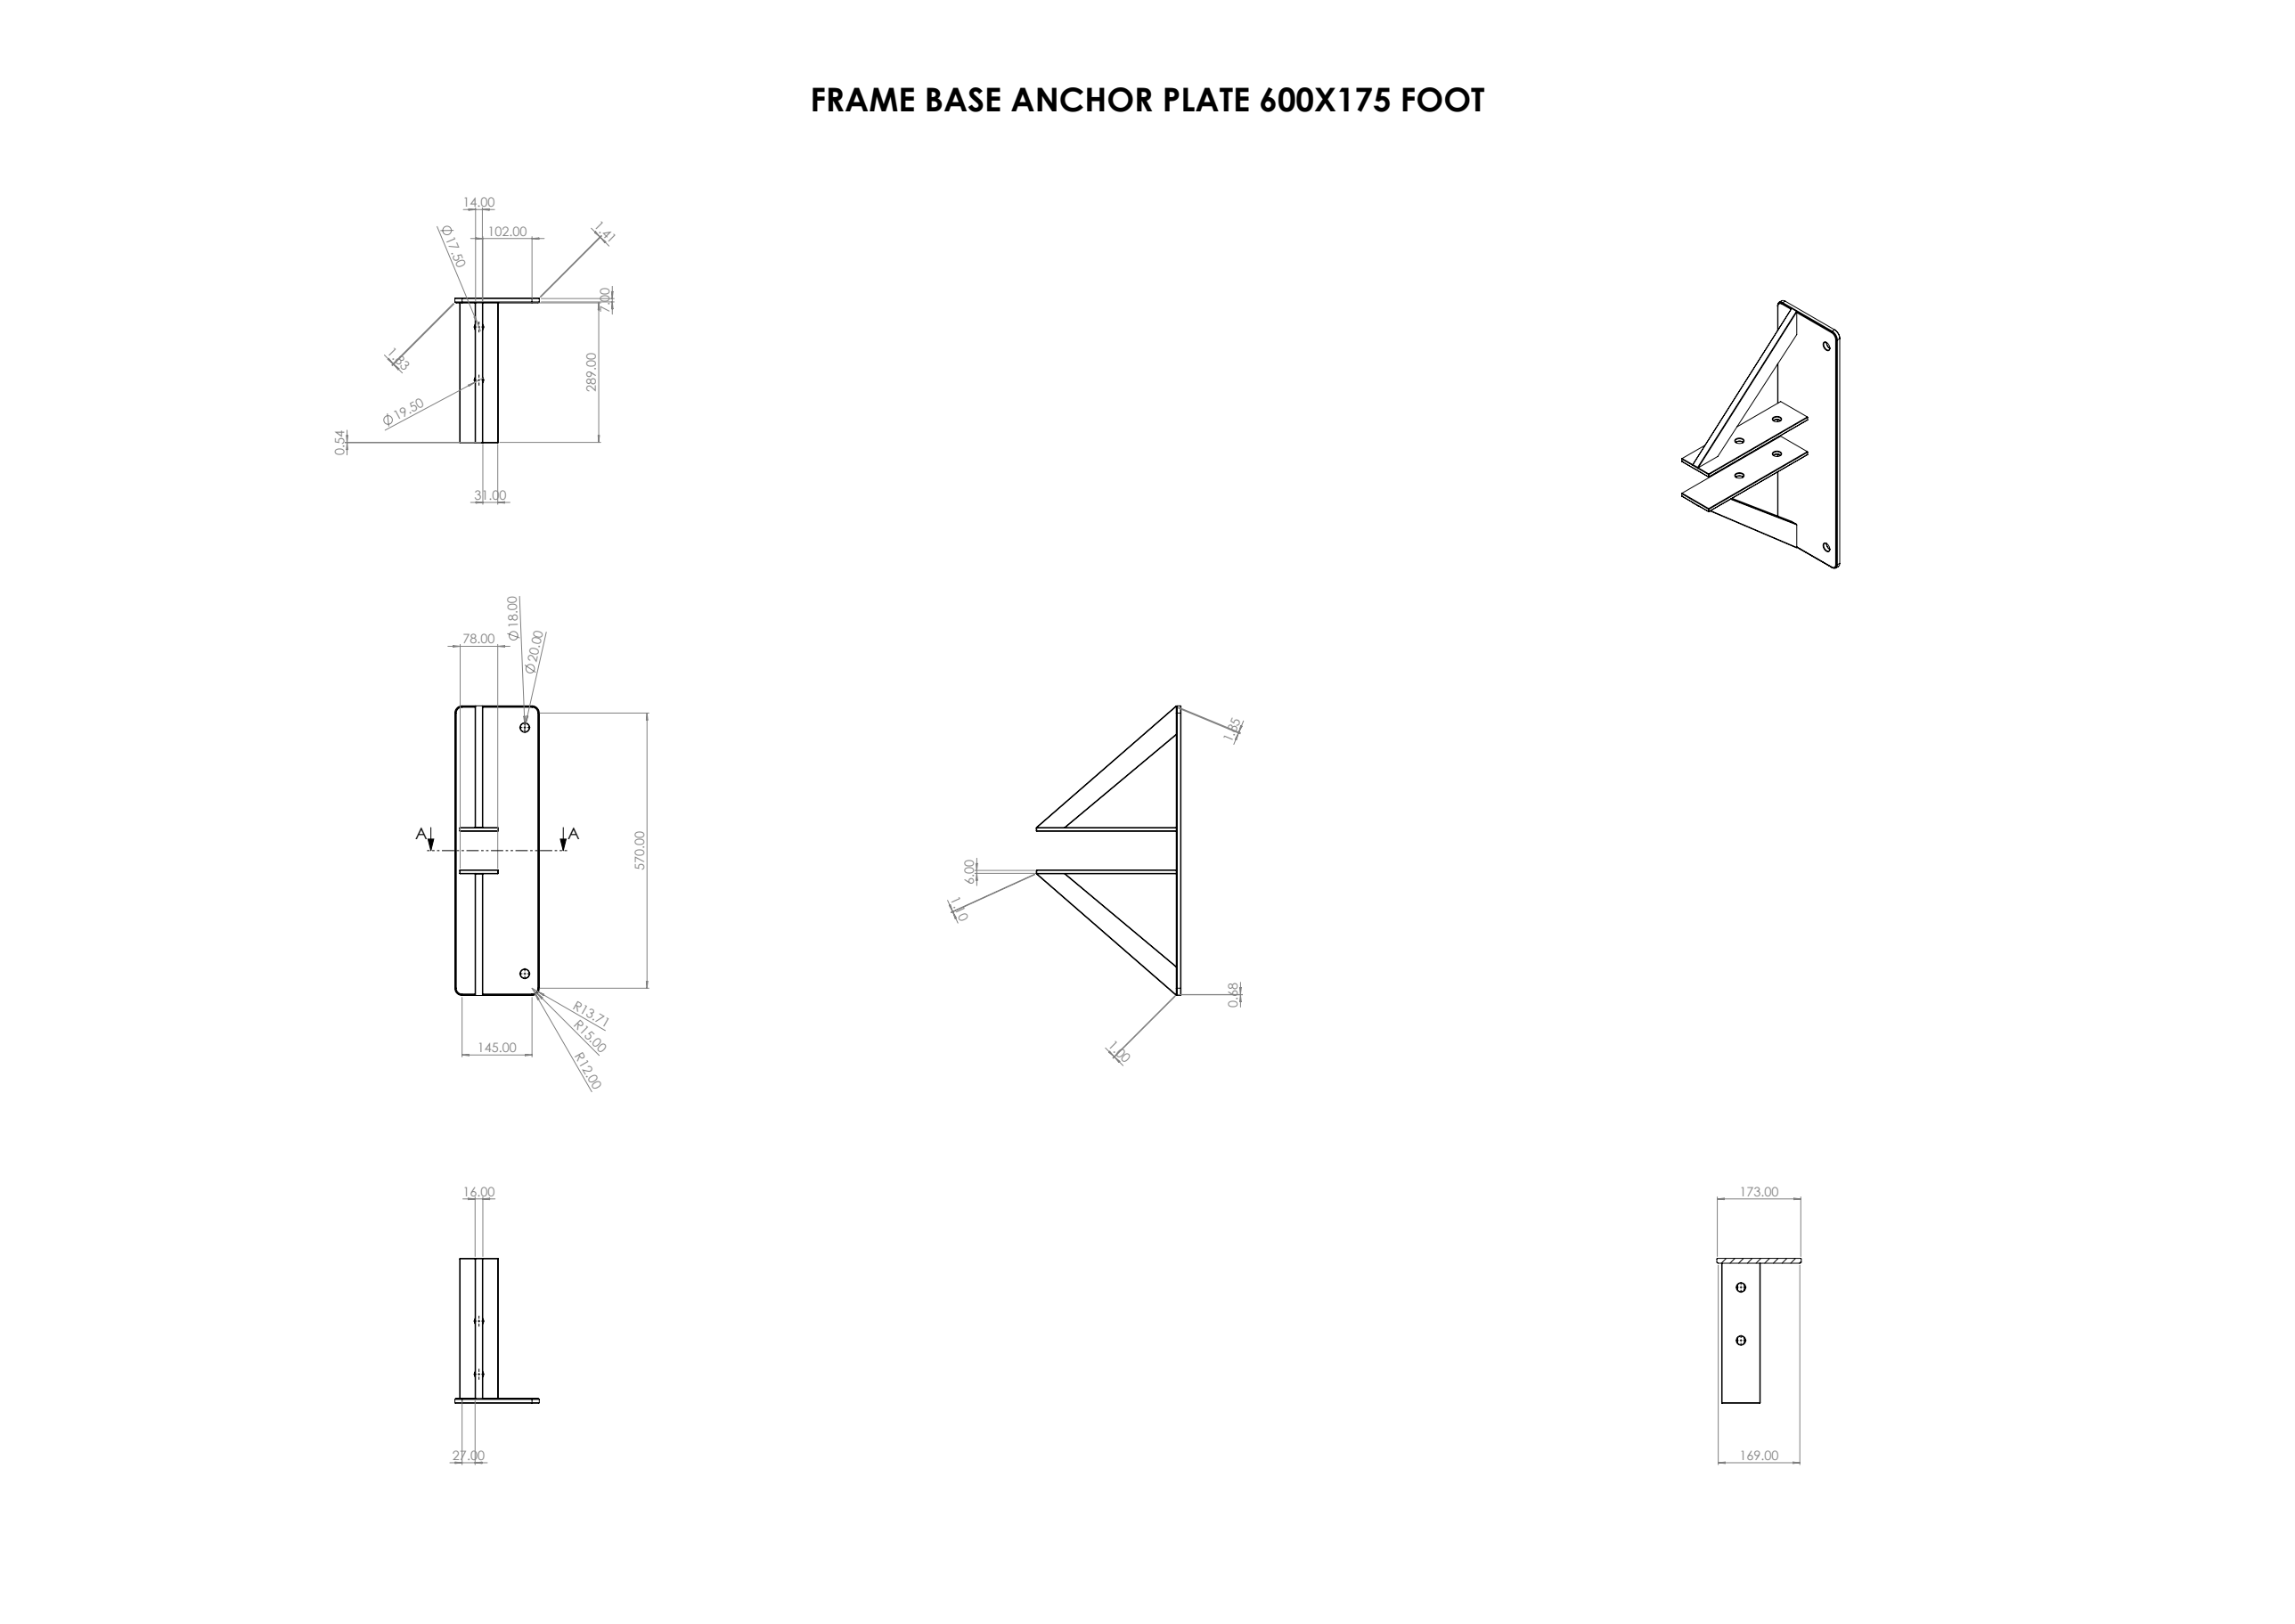
ISO-10303-21;
HEADER;
/* Generated by software containing ST-Developer
 * from STEP Tools, Inc. (www.steptools.com) 
 */

FILE_DESCRIPTION(
/* description */ (''),
/* implementation_level */ '2;1');

FILE_NAME(
/* name */ '07_Frame_Base_Anchor_Plate_600x175_Foot.step',
/* time_stamp */ '2026-10-20T10:03:03-07:00',
/* author */ (''),
/* organization */ (''),
/* preprocessor_version */ 'ST-DEVELOPER v20.2',
/* originating_system */ 'Autodesk Translation Framework v15.15.0.0',
/* authorisation */ '');

FILE_SCHEMA (('AUTOMOTIVE_DESIGN { 1 0 10303 214 3 1 1 }'));
ENDSEC;

DATA;
#10=MECHANICAL_DESIGN_GEOMETRIC_PRESENTATION_REPRESENTATION('',(#535),#71492);
#392=SHAPE_REPRESENTATION_RELATIONSHIP('SRR','None',#71613,#411);
#411=ADVANCED_BREP_SHAPE_REPRESENTATION('',(#430),#71483);
#430=MANIFOLD_SOLID_BREP('Foot',#28469);
#535=STYLED_ITEM('',(#71866),#430);
#1672=CYLINDRICAL_SURFACE('',#30065,1.5);
#1673=CYLINDRICAL_SURFACE('',#30068,1.5);
#1674=CYLINDRICAL_SURFACE('',#30093,0.875);
#1675=CYLINDRICAL_SURFACE('',#30100,0.875);
#1676=CYLINDRICAL_SURFACE('',#30108,0.875);
#1677=CYLINDRICAL_SURFACE('',#30113,0.875);
#1678=CYLINDRICAL_SURFACE('',#30118,0.899999999999999);
#1679=CYLINDRICAL_SURFACE('',#30122,0.899999999999999);
#1680=CYLINDRICAL_SURFACE('',#30161,1.5);
#1681=CYLINDRICAL_SURFACE('',#30163,1.5);
#1953=FACE_BOUND('',#5670,.T.);
#1954=FACE_BOUND('',#5671,.T.);
#1955=FACE_BOUND('',#5677,.T.);
#1956=FACE_BOUND('',#5678,.T.);
#1957=FACE_BOUND('',#5684,.T.);
#1958=FACE_BOUND('',#5685,.T.);
#1959=FACE_BOUND('',#5692,.T.);
#1960=FACE_BOUND('',#5693,.T.);
#1961=FACE_BOUND('',#5699,.T.);
#1962=FACE_BOUND('',#5700,.T.);
#1963=FACE_BOUND('',#5717,.T.);
#1964=FACE_BOUND('',#5718,.T.);
#1965=FACE_BOUND('',#5719,.T.);
#1966=FACE_BOUND('',#5720,.T.);
#2479=CIRCLE('',#30049,1.5);
#2480=CIRCLE('',#30050,1.4);
#2481=CIRCLE('',#30053,1.5);
#2482=CIRCLE('',#30054,1.4);
#2483=CIRCLE('',#30057,1.5);
#2484=CIRCLE('',#30058,1.4);
#2485=CIRCLE('',#30061,1.5);
#2486=CIRCLE('',#30062,1.4);
#2487=CIRCLE('',#30066,1.5);
#2488=CIRCLE('',#30069,1.5);
#2489=CIRCLE('',#30071,1.);
#2490=CIRCLE('',#30072,1.);
#2491=CIRCLE('',#30078,0.975000000000001);
#2492=CIRCLE('',#30079,0.975000000000001);
#2493=CIRCLE('',#30085,0.975000000000001);
#2494=CIRCLE('',#30086,0.975000000000001);
#2495=CIRCLE('',#30091,0.975000000000001);
#2496=CIRCLE('',#30092,0.875);
#2497=CIRCLE('',#30094,0.875);
#2498=CIRCLE('',#30096,0.975000000000001);
#2499=CIRCLE('',#30099,0.875);
#2500=CIRCLE('',#30101,0.875);
#2501=CIRCLE('',#30103,0.975000000000001);
#2502=CIRCLE('',#30105,0.975000000000001);
#2503=CIRCLE('',#30107,0.875);
#2504=CIRCLE('',#30109,0.875);
#2505=CIRCLE('',#30112,0.875);
#2506=CIRCLE('',#30114,0.875);
#2507=CIRCLE('',#30117,0.899999999999999);
#2508=CIRCLE('',#30119,0.899999999999999);
#2509=CIRCLE('',#30121,0.899999999999999);
#2510=CIRCLE('',#30123,0.899999999999999);
#2511=CIRCLE('',#30126,1.37071067811866);
#2512=CIRCLE('',#30127,1.2);
#2513=CIRCLE('',#30130,1.37071067811866);
#2514=CIRCLE('',#30131,1.2);
#2515=CIRCLE('',#30134,1.2);
#2516=CIRCLE('',#30135,1.2);
#2517=CIRCLE('',#30136,1.);
#2518=CIRCLE('',#30137,1.);
#2519=CIRCLE('',#30140,1.37071067811866);
#2520=CIRCLE('',#30143,1.37071067811866);
#2521=CIRCLE('',#30155,1.5);
#2522=CIRCLE('',#30158,1.5);
#2865=CONICAL_SURFACE('',#30048,1.45,0.785398163397448);
#2866=CONICAL_SURFACE('',#30052,1.45,0.78539816339746);
#2867=CONICAL_SURFACE('',#30056,1.45,0.78539816339746);
#2868=CONICAL_SURFACE('',#30060,1.45,0.785398163397448);
#2869=CONICAL_SURFACE('',#30090,0.925000000000001,0.785398163397457);
#2870=CONICAL_SURFACE('',#30097,0.925000000000001,0.785398163397457);
#2871=CONICAL_SURFACE('',#30098,0.925000000000001,0.785398163397457);
#2872=CONICAL_SURFACE('',#30102,0.925000000000001,0.785398163397457);
#2873=CONICAL_SURFACE('',#30106,0.925000000000001,0.785398163397457);
#2874=CONICAL_SURFACE('',#30110,0.925000000000001,0.785398163397457);
#2875=CONICAL_SURFACE('',#30111,0.925000000000001,0.785398163397457);
#2876=CONICAL_SURFACE('',#30115,0.925000000000001,0.785398163397457);
#2877=CONICAL_SURFACE('',#30116,0.949999999999999,0.785398163397455);
#2878=CONICAL_SURFACE('',#30120,0.949999999999999,0.785398163397455);
#2879=CONICAL_SURFACE('',#30125,1.28535533905933,1.17809724509618);
#2880=CONICAL_SURFACE('',#30129,1.28535533905933,1.17809724509618);
#2881=CONICAL_SURFACE('',#30139,1.28535533905933,1.17809724509618);
#2882=CONICAL_SURFACE('',#30142,1.28535533905933,1.17809724509618);
#2883=CONICAL_SURFACE('',#30145,0.949999999999999,0.785398163397455);
#2884=CONICAL_SURFACE('',#30146,0.949999999999999,0.785398163397455);
#2885=CONICAL_SURFACE('',#30150,1.4,0.785398163397448);
#2886=CONICAL_SURFACE('',#30152,1.4,0.785398163397448);
#2887=CONICAL_SURFACE('',#30154,1.4,0.785398163397448);
#2888=CONICAL_SURFACE('',#30157,1.4,0.785398163397448);
#3964=FACE_OUTER_BOUND('',#5623,.T.);
#3965=FACE_OUTER_BOUND('',#5624,.T.);
#3966=FACE_OUTER_BOUND('',#5625,.T.);
#3967=FACE_OUTER_BOUND('',#5626,.T.);
#3968=FACE_OUTER_BOUND('',#5627,.T.);
#3969=FACE_OUTER_BOUND('',#5628,.T.);
#3970=FACE_OUTER_BOUND('',#5629,.T.);
#3971=FACE_OUTER_BOUND('',#5630,.T.);
#3972=FACE_OUTER_BOUND('',#5631,.T.);
#3973=FACE_OUTER_BOUND('',#5632,.T.);
#3974=FACE_OUTER_BOUND('',#5633,.T.);
#3975=FACE_OUTER_BOUND('',#5634,.T.);
#3976=FACE_OUTER_BOUND('',#5635,.T.);
#3977=FACE_OUTER_BOUND('',#5636,.T.);
#3978=FACE_OUTER_BOUND('',#5637,.T.);
#3979=FACE_OUTER_BOUND('',#5638,.T.);
#3980=FACE_OUTER_BOUND('',#5639,.T.);
#3981=FACE_OUTER_BOUND('',#5640,.T.);
#3982=FACE_OUTER_BOUND('',#5641,.T.);
#3983=FACE_OUTER_BOUND('',#5642,.T.);
#3984=FACE_OUTER_BOUND('',#5643,.T.);
#3985=FACE_OUTER_BOUND('',#5644,.T.);
#3986=FACE_OUTER_BOUND('',#5645,.T.);
#3987=FACE_OUTER_BOUND('',#5646,.T.);
#3988=FACE_OUTER_BOUND('',#5647,.T.);
#3989=FACE_OUTER_BOUND('',#5648,.T.);
#3990=FACE_OUTER_BOUND('',#5649,.T.);
#3991=FACE_OUTER_BOUND('',#5650,.T.);
#3992=FACE_OUTER_BOUND('',#5651,.T.);
#3993=FACE_OUTER_BOUND('',#5652,.T.);
#3994=FACE_OUTER_BOUND('',#5653,.T.);
#3995=FACE_OUTER_BOUND('',#5654,.T.);
#3996=FACE_OUTER_BOUND('',#5655,.T.);
#3997=FACE_OUTER_BOUND('',#5656,.T.);
#3998=FACE_OUTER_BOUND('',#5657,.T.);
#3999=FACE_OUTER_BOUND('',#5658,.T.);
#4000=FACE_OUTER_BOUND('',#5659,.T.);
#4001=FACE_OUTER_BOUND('',#5660,.T.);
#4002=FACE_OUTER_BOUND('',#5661,.T.);
#4003=FACE_OUTER_BOUND('',#5662,.T.);
#4004=FACE_OUTER_BOUND('',#5663,.T.);
#4005=FACE_OUTER_BOUND('',#5664,.T.);
#4006=FACE_OUTER_BOUND('',#5665,.T.);
#4007=FACE_OUTER_BOUND('',#5666,.T.);
#4008=FACE_OUTER_BOUND('',#5667,.T.);
#4009=FACE_OUTER_BOUND('',#5668,.T.);
#4010=FACE_OUTER_BOUND('',#5669,.T.);
#4011=FACE_OUTER_BOUND('',#5672,.T.);
#4012=FACE_OUTER_BOUND('',#5673,.T.);
#4013=FACE_OUTER_BOUND('',#5674,.T.);
#4014=FACE_OUTER_BOUND('',#5675,.T.);
#4015=FACE_OUTER_BOUND('',#5676,.T.);
#4016=FACE_OUTER_BOUND('',#5679,.T.);
#4017=FACE_OUTER_BOUND('',#5680,.T.);
#4018=FACE_OUTER_BOUND('',#5681,.T.);
#4019=FACE_OUTER_BOUND('',#5682,.T.);
#4020=FACE_OUTER_BOUND('',#5683,.T.);
#4021=FACE_OUTER_BOUND('',#5686,.T.);
#4022=FACE_OUTER_BOUND('',#5687,.T.);
#4023=FACE_OUTER_BOUND('',#5688,.T.);
#4024=FACE_OUTER_BOUND('',#5689,.T.);
#4025=FACE_OUTER_BOUND('',#5690,.T.);
#4026=FACE_OUTER_BOUND('',#5691,.T.);
#4027=FACE_OUTER_BOUND('',#5694,.T.);
#4028=FACE_OUTER_BOUND('',#5695,.T.);
#4029=FACE_OUTER_BOUND('',#5696,.T.);
#4030=FACE_OUTER_BOUND('',#5697,.T.);
#4031=FACE_OUTER_BOUND('',#5698,.T.);
#4032=FACE_OUTER_BOUND('',#5701,.T.);
#4033=FACE_OUTER_BOUND('',#5702,.T.);
#4034=FACE_OUTER_BOUND('',#5703,.T.);
#4035=FACE_OUTER_BOUND('',#5704,.T.);
#4036=FACE_OUTER_BOUND('',#5705,.T.);
#4037=FACE_OUTER_BOUND('',#5706,.T.);
#4038=FACE_OUTER_BOUND('',#5707,.T.);
#4039=FACE_OUTER_BOUND('',#5708,.T.);
#4040=FACE_OUTER_BOUND('',#5709,.T.);
#4041=FACE_OUTER_BOUND('',#5710,.T.);
#4042=FACE_OUTER_BOUND('',#5711,.T.);
#4043=FACE_OUTER_BOUND('',#5712,.T.);
#4044=FACE_OUTER_BOUND('',#5713,.T.);
#4045=FACE_OUTER_BOUND('',#5714,.T.);
#4046=FACE_OUTER_BOUND('',#5715,.T.);
#4047=FACE_OUTER_BOUND('',#5716,.T.);
#4048=FACE_OUTER_BOUND('',#5721,.T.);
#4049=FACE_OUTER_BOUND('',#5722,.T.);
#4050=FACE_OUTER_BOUND('',#5723,.T.);
#4051=FACE_OUTER_BOUND('',#5724,.T.);
#4052=FACE_OUTER_BOUND('',#5725,.T.);
#4053=FACE_OUTER_BOUND('',#5726,.T.);
#4054=FACE_OUTER_BOUND('',#5727,.T.);
#4055=FACE_OUTER_BOUND('',#5728,.T.);
#4056=FACE_OUTER_BOUND('',#5729,.T.);
#4057=FACE_OUTER_BOUND('',#5730,.T.);
#4058=FACE_OUTER_BOUND('',#5731,.T.);
#4059=FACE_OUTER_BOUND('',#5732,.T.);
#4060=FACE_OUTER_BOUND('',#5733,.T.);
#4061=FACE_OUTER_BOUND('',#5734,.T.);
#4062=FACE_OUTER_BOUND('',#5735,.T.);
#4063=FACE_OUTER_BOUND('',#5736,.T.);
#4064=FACE_OUTER_BOUND('',#5737,.T.);
#4065=FACE_OUTER_BOUND('',#5738,.T.);
#4066=FACE_OUTER_BOUND('',#5739,.T.);
#4067=FACE_OUTER_BOUND('',#5740,.T.);
#4068=FACE_OUTER_BOUND('',#5741,.T.);
#4069=FACE_OUTER_BOUND('',#5742,.T.);
#5623=EDGE_LOOP('',(#23045,#23046,#23047,#23048));
#5624=EDGE_LOOP('',(#23049,#23050,#23051,#23052));
#5625=EDGE_LOOP('',(#23053,#23054,#23055,#23056));
#5626=EDGE_LOOP('',(#23057,#23058,#23059,#23060));
#5627=EDGE_LOOP('',(#23061,#23062,#23063,#23064));
#5628=EDGE_LOOP('',(#23065,#23066,#23067,#23068));
#5629=EDGE_LOOP('',(#23069,#23070,#23071,#23072,#23073));
#5630=EDGE_LOOP('',(#23074,#23075,#23076,#23077,#23078,#23079,#23080,#23081));
#5631=EDGE_LOOP('',(#23082,#23083,#23084));
#5632=EDGE_LOOP('',(#23085,#23086,#23087,#23088,#23089));
#5633=EDGE_LOOP('',(#23090,#23091,#23092));
#5634=EDGE_LOOP('',(#23093,#23094,#23095,#23096,#23097,#23098,#23099));
#5635=EDGE_LOOP('',(#23100,#23101,#23102,#23103,#23104,#23105));
#5636=EDGE_LOOP('',(#23106,#23107,#23108,#23109,#23110,#23111));
#5637=EDGE_LOOP('',(#23112,#23113,#23114,#23115,#23116,#23117));
#5638=EDGE_LOOP('',(#23118,#23119,#23120,#23121,#23122));
#5639=EDGE_LOOP('',(#23123,#23124,#23125,#23126,#23127,#23128));
#5640=EDGE_LOOP('',(#23129,#23130,#23131,#23132,#23133));
#5641=EDGE_LOOP('',(#23134,#23135,#23136,#23137,#23138));
#5642=EDGE_LOOP('',(#23139,#23140,#23141,#23142,#23143));
#5643=EDGE_LOOP('',(#23144,#23145,#23146,#23147,#23148,#23149,#23150,#23151));
#5644=EDGE_LOOP('',(#23152,#23153,#23154,#23155));
#5645=EDGE_LOOP('',(#23156,#23157,#23158,#23159,#23160,#23161,#23162));
#5646=EDGE_LOOP('',(#23163,#23164,#23165,#23166,#23167,#23168));
#5647=EDGE_LOOP('',(#23169,#23170,#23171,#23172,#23173));
#5648=EDGE_LOOP('',(#23174,#23175,#23176,#23177,#23178,#23179,#23180));
#5649=EDGE_LOOP('',(#23181,#23182,#23183));
#5650=EDGE_LOOP('',(#23184,#23185,#23186));
#5651=EDGE_LOOP('',(#23187,#23188,#23189,#23190,#23191,#23192));
#5652=EDGE_LOOP('',(#23193,#23194,#23195,#23196,#23197,#23198));
#5653=EDGE_LOOP('',(#23199,#23200,#23201,#23202,#23203));
#5654=EDGE_LOOP('',(#23204,#23205,#23206,#23207,#23208,#23209));
#5655=EDGE_LOOP('',(#23210,#23211,#23212,#23213,#23214,#23215));
#5656=EDGE_LOOP('',(#23216,#23217,#23218,#23219,#23220));
#5657=EDGE_LOOP('',(#23221,#23222,#23223,#23224));
#5658=EDGE_LOOP('',(#23225,#23226,#23227,#23228));
#5659=EDGE_LOOP('',(#23229,#23230,#23231,#23232));
#5660=EDGE_LOOP('',(#23233,#23234,#23235,#23236));
#5661=EDGE_LOOP('',(#23237,#23238,#23239,#23240));
#5662=EDGE_LOOP('',(#23241,#23242,#23243,#23244));
#5663=EDGE_LOOP('',(#23245,#23246,#23247,#23248));
#5664=EDGE_LOOP('',(#23249,#23250,#23251,#23252));
#5665=EDGE_LOOP('',(#23253,#23254,#23255,#23256));
#5666=EDGE_LOOP('',(#23257,#23258,#23259,#23260));
#5667=EDGE_LOOP('',(#23261,#23262,#23263,#23264));
#5668=EDGE_LOOP('',(#23265,#23266,#23267,#23268));
#5669=EDGE_LOOP('',(#23269,#23270,#23271,#23272,#23273,#23274,#23275,#23276));
#5670=EDGE_LOOP('',(#23277));
#5671=EDGE_LOOP('',(#23278));
#5672=EDGE_LOOP('',(#23279,#23280,#23281,#23282));
#5673=EDGE_LOOP('',(#23283,#23284,#23285,#23286));
#5674=EDGE_LOOP('',(#23287,#23288,#23289,#23290,#23291));
#5675=EDGE_LOOP('',(#23292,#23293,#23294,#23295,#23296));
#5676=EDGE_LOOP('',(#23297,#23298,#23299,#23300,#23301,#23302,#23303,#23304,
#23305,#23306,#23307,#23308,#23309,#23310,#23311,#23312));
#5677=EDGE_LOOP('',(#23313));
#5678=EDGE_LOOP('',(#23314));
#5679=EDGE_LOOP('',(#23315,#23316,#23317,#23318,#23319));
#5680=EDGE_LOOP('',(#23320,#23321,#23322,#23323,#23324));
#5681=EDGE_LOOP('',(#23325,#23326,#23327,#23328,#23329));
#5682=EDGE_LOOP('',(#23330,#23331,#23332,#23333,#23334));
#5683=EDGE_LOOP('',(#23335,#23336,#23337,#23338,#23339,#23340,#23341,#23342,
#23343,#23344,#23345,#23346,#23347,#23348,#23349,#23350));
#5684=EDGE_LOOP('',(#23351));
#5685=EDGE_LOOP('',(#23352));
#5686=EDGE_LOOP('',(#23353,#23354,#23355,#23356));
#5687=EDGE_LOOP('',(#23357,#23358,#23359,#23360,#23361));
#5688=EDGE_LOOP('',(#23362,#23363,#23364,#23365));
#5689=EDGE_LOOP('',(#23366,#23367,#23368,#23369));
#5690=EDGE_LOOP('',(#23370,#23371,#23372,#23373));
#5691=EDGE_LOOP('',(#23374,#23375,#23376,#23377));
#5692=EDGE_LOOP('',(#23378));
#5693=EDGE_LOOP('',(#23379));
#5694=EDGE_LOOP('',(#23380,#23381,#23382,#23383));
#5695=EDGE_LOOP('',(#23384,#23385,#23386,#23387));
#5696=EDGE_LOOP('',(#23388,#23389,#23390,#23391));
#5697=EDGE_LOOP('',(#23392,#23393,#23394,#23395));
#5698=EDGE_LOOP('',(#23396,#23397,#23398,#23399));
#5699=EDGE_LOOP('',(#23400));
#5700=EDGE_LOOP('',(#23401));
#5701=EDGE_LOOP('',(#23402,#23403,#23404,#23405));
#5702=EDGE_LOOP('',(#23406,#23407,#23408,#23409));
#5703=EDGE_LOOP('',(#23410,#23411,#23412,#23413));
#5704=EDGE_LOOP('',(#23414,#23415,#23416,#23417));
#5705=EDGE_LOOP('',(#23418,#23419,#23420,#23421));
#5706=EDGE_LOOP('',(#23422,#23423,#23424,#23425));
#5707=EDGE_LOOP('',(#23426,#23427,#23428,#23429));
#5708=EDGE_LOOP('',(#23430,#23431,#23432,#23433));
#5709=EDGE_LOOP('',(#23434,#23435,#23436,#23437));
#5710=EDGE_LOOP('',(#23438,#23439,#23440,#23441));
#5711=EDGE_LOOP('',(#23442,#23443,#23444,#23445));
#5712=EDGE_LOOP('',(#23446,#23447,#23448,#23449));
#5713=EDGE_LOOP('',(#23450,#23451,#23452,#23453));
#5714=EDGE_LOOP('',(#23454,#23455,#23456,#23457));
#5715=EDGE_LOOP('',(#23458,#23459,#23460,#23461));
#5716=EDGE_LOOP('',(#23462,#23463,#23464,#23465,#23466,#23467,#23468,#23469,
#23470,#23471,#23472,#23473,#23474,#23475,#23476,#23477,#23478,#23479,#23480,
#23481));
#5717=EDGE_LOOP('',(#23482));
#5718=EDGE_LOOP('',(#23483,#23484,#23485,#23486,#23487,#23488,#23489,#23490));
#5719=EDGE_LOOP('',(#23491,#23492,#23493,#23494,#23495,#23496,#23497,#23498));
#5720=EDGE_LOOP('',(#23499));
#5721=EDGE_LOOP('',(#23500,#23501,#23502,#23503));
#5722=EDGE_LOOP('',(#23504,#23505,#23506,#23507));
#5723=EDGE_LOOP('',(#23508,#23509,#23510,#23511));
#5724=EDGE_LOOP('',(#23512,#23513,#23514,#23515));
#5725=EDGE_LOOP('',(#23516,#23517,#23518,#23519));
#5726=EDGE_LOOP('',(#23520,#23521,#23522,#23523));
#5727=EDGE_LOOP('',(#23524,#23525,#23526,#23527));
#5728=EDGE_LOOP('',(#23528,#23529,#23530,#23531));
#5729=EDGE_LOOP('',(#23532,#23533,#23534,#23535,#23536,#23537));
#5730=EDGE_LOOP('',(#23538,#23539,#23540,#23541,#23542,#23543,#23544));
#5731=EDGE_LOOP('',(#23545,#23546,#23547,#23548));
#5732=EDGE_LOOP('',(#23549,#23550,#23551,#23552));
#5733=EDGE_LOOP('',(#23553,#23554,#23555,#23556));
#5734=EDGE_LOOP('',(#23557,#23558,#23559,#23560,#23561,#23562,#23563,#23564));
#5735=EDGE_LOOP('',(#23565,#23566,#23567,#23568));
#5736=EDGE_LOOP('',(#23569,#23570,#23571,#23572));
#5737=EDGE_LOOP('',(#23573,#23574,#23575,#23576));
#5738=EDGE_LOOP('',(#23577,#23578,#23579,#23580,#23581,#23582,#23583,#23584));
#5739=EDGE_LOOP('',(#23585,#23586,#23587,#23588));
#5740=EDGE_LOOP('',(#23589,#23590,#23591,#23592));
#5741=EDGE_LOOP('',(#23593,#23594,#23595,#23596));
#5742=EDGE_LOOP('',(#23597,#23598,#23599,#23600));
#8008=LINE('',#50006,#10496);
#8009=LINE('',#50008,#10497);
#8010=LINE('',#50010,#10498);
#8011=LINE('',#50011,#10499);
#8012=LINE('',#50014,#10500);
#8013=LINE('',#50016,#10501);
#8014=LINE('',#50017,#10502);
#8015=LINE('',#50020,#10503);
#8016=LINE('',#50022,#10504);
#8017=LINE('',#50023,#10505);
#8018=LINE('',#50027,#10506);
#8019=LINE('',#50029,#10507);
#8020=LINE('',#50031,#10508);
#8021=LINE('',#50032,#10509);
#8022=LINE('',#50035,#10510);
#8023=LINE('',#50037,#10511);
#8024=LINE('',#50038,#10512);
#8025=LINE('',#50041,#10513);
#8026=LINE('',#50043,#10514);
#8027=LINE('',#50044,#10515);
#8028=LINE('',#50048,#10516);
#8029=LINE('',#50050,#10517);
#8030=LINE('',#50052,#10518);
#8031=LINE('',#50054,#10519);
#8032=LINE('',#50055,#10520);
#8033=LINE('',#50058,#10521);
#8034=LINE('',#50060,#10522);
#8035=LINE('',#50062,#10523);
#8036=LINE('',#50064,#10524);
#8037=LINE('',#50066,#10525);
#8038=LINE('',#50068,#10526);
#8039=LINE('',#50069,#10527);
#8040=LINE('',#50072,#10528);
#8041=LINE('',#50073,#10529);
#8042=LINE('',#50076,#10530);
#8043=LINE('',#50078,#10531);
#8044=LINE('',#50080,#10532);
#8045=LINE('',#50081,#10533);
#8046=LINE('',#50084,#10534);
#8047=LINE('',#50085,#10535);
#8048=LINE('',#50088,#10536);
#8049=LINE('',#50090,#10537);
#8050=LINE('',#50092,#10538);
#8051=LINE('',#50093,#10539);
#8052=LINE('',#50094,#10540);
#8053=LINE('',#50097,#10541);
#8054=LINE('',#50099,#10542);
#8055=LINE('',#50101,#10543);
#8056=LINE('',#50103,#10544);
#8057=LINE('',#50104,#10545);
#8058=LINE('',#50107,#10546);
#8059=LINE('',#50109,#10547);
#8060=LINE('',#50111,#10548);
#8061=LINE('',#50113,#10549);
#8062=LINE('',#50114,#10550);
#8063=LINE('',#50117,#10551);
#8064=LINE('',#50119,#10552);
#8065=LINE('',#50121,#10553);
#8066=LINE('',#50122,#10554);
#8067=LINE('',#50125,#10555);
#8068=LINE('',#50127,#10556);
#8069=LINE('',#50128,#10557);
#8070=LINE('',#50131,#10558);
#8071=LINE('',#50133,#10559);
#8072=LINE('',#50135,#10560);
#8073=LINE('',#50136,#10561);
#8074=LINE('',#50139,#10562);
#8075=LINE('',#50140,#10563);
#8076=LINE('',#50143,#10564);
#8077=LINE('',#50145,#10565);
#8078=LINE('',#50146,#10566);
#8079=LINE('',#50150,#10567);
#8080=LINE('',#50152,#10568);
#8081=LINE('',#50154,#10569);
#8082=LINE('',#50156,#10570);
#8083=LINE('',#50157,#10571);
#8084=LINE('',#50160,#10572);
#8085=LINE('',#50162,#10573);
#8086=LINE('',#50164,#10574);
#8087=LINE('',#50166,#10575);
#8088=LINE('',#50168,#10576);
#8089=LINE('',#50170,#10577);
#8090=LINE('',#50171,#10578);
#8091=LINE('',#50174,#10579);
#8092=LINE('',#50175,#10580);
#8093=LINE('',#50178,#10581);
#8094=LINE('',#50180,#10582);
#8095=LINE('',#50182,#10583);
#8096=LINE('',#50183,#10584);
#8097=LINE('',#50184,#10585);
#8098=LINE('',#50187,#10586);
#8099=LINE('',#50189,#10587);
#8100=LINE('',#50190,#10588);
#8101=LINE('',#50193,#10589);
#8102=LINE('',#50194,#10590);
#8103=LINE('',#50196,#10591);
#8104=LINE('',#50198,#10592);
#8105=LINE('',#50200,#10593);
#8106=LINE('',#50201,#10594);
#8107=LINE('',#50204,#10595);
#8108=LINE('',#50205,#10596);
#8109=LINE('',#50208,#10597);
#8110=LINE('',#50209,#10598);
#8111=LINE('',#50212,#10599);
#8112=LINE('',#50214,#10600);
#8113=LINE('',#50216,#10601);
#8114=LINE('',#50218,#10602);
#8115=LINE('',#50219,#10603);
#8116=LINE('',#50222,#10604);
#8117=LINE('',#50224,#10605);
#8118=LINE('',#50226,#10606);
#8119=LINE('',#50228,#10607);
#8120=LINE('',#50229,#10608);
#8121=LINE('',#50232,#10609);
#8122=LINE('',#50234,#10610);
#8123=LINE('',#50236,#10611);
#8124=LINE('',#50237,#10612);
#8125=LINE('',#50240,#10613);
#8126=LINE('',#50242,#10614);
#8127=LINE('',#50243,#10615);
#8128=LINE('',#50246,#10616);
#8129=LINE('',#50248,#10617);
#8130=LINE('',#50250,#10618);
#8131=LINE('',#50251,#10619);
#8132=LINE('',#50254,#10620);
#8133=LINE('',#50256,#10621);
#8134=LINE('',#50257,#10622);
#8135=LINE('',#50261,#10623);
#8136=LINE('',#50265,#10624);
#8137=LINE('',#50270,#10625);
#8138=LINE('',#50271,#10626);
#8139=LINE('',#50272,#10627);
#8140=LINE('',#50276,#10628);
#8141=LINE('',#50282,#10629);
#8142=LINE('',#50283,#10630);
#8143=LINE('',#50284,#10631);
#8144=LINE('',#50288,#10632);
#8145=LINE('',#50294,#10633);
#8146=LINE('',#50295,#10634);
#8147=LINE('',#50296,#10635);
#8148=LINE('',#50300,#10636);
#8149=LINE('',#50304,#10637);
#8150=LINE('',#50305,#10638);
#8151=LINE('',#50308,#10639);
#8152=LINE('',#50310,#10640);
#8153=LINE('',#50311,#10641);
#8154=LINE('',#50314,#10642);
#8155=LINE('',#50318,#10643);
#8156=LINE('',#50319,#10644);
#8157=LINE('',#50322,#10645);
#8158=LINE('',#50331,#10646);
#8159=LINE('',#50332,#10647);
#8160=LINE('',#50335,#10648);
#8161=LINE('',#50336,#10649);
#8162=LINE('',#50339,#10650);
#8163=LINE('',#50341,#10651);
#8164=LINE('',#50342,#10652);
#8165=LINE('',#50344,#10653);
#8166=LINE('',#50347,#10654);
#8167=LINE('',#50349,#10655);
#8168=LINE('',#50350,#10656);
#8169=LINE('',#50356,#10657);
#8170=LINE('',#50357,#10658);
#8171=LINE('',#50361,#10659);
#8172=LINE('',#50363,#10660);
#8173=LINE('',#50365,#10661);
#8174=LINE('',#50366,#10662);
#8175=LINE('',#50368,#10663);
#8176=LINE('',#50370,#10664);
#8177=LINE('',#50371,#10665);
#8178=LINE('',#50378,#10666);
#8179=LINE('',#50379,#10667);
#8180=LINE('',#50382,#10668);
#8181=LINE('',#50383,#10669);
#8182=LINE('',#50385,#10670);
#8183=LINE('',#50390,#10671);
#8184=LINE('',#50395,#10672);
#8185=LINE('',#50397,#10673);
#8186=LINE('',#50401,#10674);
#8187=LINE('',#50404,#10675);
#8188=LINE('',#50409,#10676);
#8189=LINE('',#50413,#10677);
#8190=LINE('',#50415,#10678);
#8191=LINE('',#50420,#10679);
#8192=LINE('',#50425,#10680);
#8193=LINE('',#50427,#10681);
#8194=LINE('',#50430,#10682);
#8195=LINE('',#50435,#10683);
#8196=LINE('',#50437,#10684);
#8197=LINE('',#50440,#10685);
#8198=LINE('',#50444,#10686);
#8199=LINE('',#50448,#10687);
#8200=LINE('',#50452,#10688);
#8201=LINE('',#50456,#10689);
#8202=LINE('',#50458,#10690);
#8203=LINE('',#50459,#10691);
#8204=LINE('',#50463,#10692);
#8205=LINE('',#50469,#10693);
#8206=LINE('',#50470,#10694);
#8207=LINE('',#50471,#10695);
#8208=LINE('',#50475,#10696);
#8209=LINE('',#50479,#10697);
#8210=LINE('',#50480,#10698);
#8211=LINE('',#50483,#10699);
#8212=LINE('',#50485,#10700);
#8213=LINE('',#50489,#10701);
#8214=LINE('',#50492,#10702);
#8215=LINE('',#50499,#10703);
#8216=LINE('',#50500,#10704);
#8217=LINE('',#50503,#10705);
#8218=LINE('',#50507,#10706);
#8219=LINE('',#50508,#10707);
#8220=LINE('',#50511,#10708);
#8221=LINE('',#50515,#10709);
#8222=LINE('',#50516,#10710);
#8223=LINE('',#50518,#10711);
#8224=LINE('',#50520,#10712);
#8225=LINE('',#50522,#10713);
#8226=LINE('',#50525,#10714);
#8227=LINE('',#50526,#10715);
#8228=LINE('',#50528,#10716);
#8229=LINE('',#50530,#10717);
#8230=LINE('',#50531,#10718);
#8231=LINE('',#50533,#10719);
#8232=LINE('',#50535,#10720);
#8233=LINE('',#50537,#10721);
#8234=LINE('',#50540,#10722);
#8235=LINE('',#50544,#10723);
#8236=LINE('',#50545,#10724);
#8237=LINE('',#50548,#10725);
#8238=LINE('',#50551,#10726);
#8239=LINE('',#50553,#10727);
#8240=LINE('',#50554,#10728);
#8241=LINE('',#50556,#10729);
#10496=VECTOR('',#35215,1.);
#10497=VECTOR('',#35216,1.);
#10498=VECTOR('',#35217,1.);
#10499=VECTOR('',#35218,1.);
#10500=VECTOR('',#35221,1.);
#10501=VECTOR('',#35222,1.);
#10502=VECTOR('',#35223,1.);
#10503=VECTOR('',#35226,1.);
#10504=VECTOR('',#35227,1.);
#10505=VECTOR('',#35228,1.);
#10506=VECTOR('',#35231,1.);
#10507=VECTOR('',#35232,1.);
#10508=VECTOR('',#35233,1.);
#10509=VECTOR('',#35234,1.);
#10510=VECTOR('',#35237,1.);
#10511=VECTOR('',#35238,1.);
#10512=VECTOR('',#35239,1.);
#10513=VECTOR('',#35242,1.);
#10514=VECTOR('',#35243,1.);
#10515=VECTOR('',#35244,1.);
#10516=VECTOR('',#35247,1.);
#10517=VECTOR('',#35248,1.);
#10518=VECTOR('',#35249,1.);
#10519=VECTOR('',#35250,1.);
#10520=VECTOR('',#35251,1.);
#10521=VECTOR('',#35254,1.);
#10522=VECTOR('',#35255,1.);
#10523=VECTOR('',#35256,1.);
#10524=VECTOR('',#35257,1.);
#10525=VECTOR('',#35258,1.);
#10526=VECTOR('',#35259,1.);
#10527=VECTOR('',#35260,1.);
#10528=VECTOR('',#35263,1.);
#10529=VECTOR('',#35264,1.);
#10530=VECTOR('',#35267,1.);
#10531=VECTOR('',#35268,1.);
#10532=VECTOR('',#35269,1.);
#10533=VECTOR('',#35270,1.);
#10534=VECTOR('',#35273,1.);
#10535=VECTOR('',#35274,1.);
#10536=VECTOR('',#35277,1.);
#10537=VECTOR('',#35278,1.);
#10538=VECTOR('',#35279,1.);
#10539=VECTOR('',#35280,1.);
#10540=VECTOR('',#35281,1.);
#10541=VECTOR('',#35284,1.);
#10542=VECTOR('',#35285,1.);
#10543=VECTOR('',#35286,1.);
#10544=VECTOR('',#35287,1.);
#10545=VECTOR('',#35288,1.);
#10546=VECTOR('',#35291,1.);
#10547=VECTOR('',#35292,1.);
#10548=VECTOR('',#35293,1.);
#10549=VECTOR('',#35294,1.);
#10550=VECTOR('',#35295,1.);
#10551=VECTOR('',#35298,1.);
#10552=VECTOR('',#35299,1.);
#10553=VECTOR('',#35300,1.);
#10554=VECTOR('',#35301,1.);
#10555=VECTOR('',#35304,1.);
#10556=VECTOR('',#35305,1.);
#10557=VECTOR('',#35306,1.);
#10558=VECTOR('',#35309,1.);
#10559=VECTOR('',#35310,1.);
#10560=VECTOR('',#35311,1.);
#10561=VECTOR('',#35312,1.);
#10562=VECTOR('',#35315,1.);
#10563=VECTOR('',#35316,1.);
#10564=VECTOR('',#35319,1.);
#10565=VECTOR('',#35320,1.);
#10566=VECTOR('',#35321,1.);
#10567=VECTOR('',#35324,1.);
#10568=VECTOR('',#35325,1.);
#10569=VECTOR('',#35326,1.);
#10570=VECTOR('',#35327,1.);
#10571=VECTOR('',#35328,1.);
#10572=VECTOR('',#35331,1.);
#10573=VECTOR('',#35332,1.);
#10574=VECTOR('',#35333,1.);
#10575=VECTOR('',#35334,1.);
#10576=VECTOR('',#35335,1.);
#10577=VECTOR('',#35336,1.);
#10578=VECTOR('',#35337,1.);
#10579=VECTOR('',#35340,1.);
#10580=VECTOR('',#35341,1.);
#10581=VECTOR('',#35344,1.);
#10582=VECTOR('',#35345,1.);
#10583=VECTOR('',#35346,1.);
#10584=VECTOR('',#35347,1.);
#10585=VECTOR('',#35348,1.);
#10586=VECTOR('',#35351,1.);
#10587=VECTOR('',#35352,1.);
#10588=VECTOR('',#35353,1.);
#10589=VECTOR('',#35356,1.);
#10590=VECTOR('',#35357,1.);
#10591=VECTOR('',#35360,1.);
#10592=VECTOR('',#35361,1.);
#10593=VECTOR('',#35362,1.);
#10594=VECTOR('',#35363,1.);
#10595=VECTOR('',#35366,1.);
#10596=VECTOR('',#35367,1.);
#10597=VECTOR('',#35370,1.);
#10598=VECTOR('',#35371,1.);
#10599=VECTOR('',#35374,1.);
#10600=VECTOR('',#35375,1.);
#10601=VECTOR('',#35376,1.);
#10602=VECTOR('',#35377,1.);
#10603=VECTOR('',#35378,1.);
#10604=VECTOR('',#35381,1.);
#10605=VECTOR('',#35382,1.);
#10606=VECTOR('',#35383,1.);
#10607=VECTOR('',#35384,1.);
#10608=VECTOR('',#35385,1.);
#10609=VECTOR('',#35388,1.);
#10610=VECTOR('',#35389,1.);
#10611=VECTOR('',#35390,1.);
#10612=VECTOR('',#35391,1.);
#10613=VECTOR('',#35394,1.);
#10614=VECTOR('',#35395,1.);
#10615=VECTOR('',#35396,1.);
#10616=VECTOR('',#35399,1.);
#10617=VECTOR('',#35400,1.);
#10618=VECTOR('',#35401,1.);
#10619=VECTOR('',#35402,1.);
#10620=VECTOR('',#35405,1.);
#10621=VECTOR('',#35406,1.);
#10622=VECTOR('',#35407,1.);
#10623=VECTOR('',#35410,1.);
#10624=VECTOR('',#35413,1.);
#10625=VECTOR('',#35418,1.);
#10626=VECTOR('',#35419,1.);
#10627=VECTOR('',#35420,1.);
#10628=VECTOR('',#35423,1.);
#10629=VECTOR('',#35430,1.);
#10630=VECTOR('',#35431,1.);
#10631=VECTOR('',#35432,1.);
#10632=VECTOR('',#35435,1.);
#10633=VECTOR('',#35442,1.);
#10634=VECTOR('',#35443,1.);
#10635=VECTOR('',#35444,1.);
#10636=VECTOR('',#35447,1.);
#10637=VECTOR('',#35454,1.);
#10638=VECTOR('',#35455,1.);
#10639=VECTOR('',#35458,1.);
#10640=VECTOR('',#35459,1.);
#10641=VECTOR('',#35460,1.);
#10642=VECTOR('',#35463,1.);
#10643=VECTOR('',#35468,1.);
#10644=VECTOR('',#35469,1.);
#10645=VECTOR('',#35472,1.);
#10646=VECTOR('',#35483,1.);
#10647=VECTOR('',#35484,1.);
#10648=VECTOR('',#35487,1.);
#10649=VECTOR('',#35488,1.);
#10650=VECTOR('',#35491,1.);
#10651=VECTOR('',#35492,1.);
#10652=VECTOR('',#35493,1.);
#10653=VECTOR('',#35496,1.);
#10654=VECTOR('',#35499,1.);
#10655=VECTOR('',#35500,1.);
#10656=VECTOR('',#35501,1.);
#10657=VECTOR('',#35508,1.);
#10658=VECTOR('',#35509,1.);
#10659=VECTOR('',#35514,1.);
#10660=VECTOR('',#35515,1.);
#10661=VECTOR('',#35516,1.);
#10662=VECTOR('',#35517,1.);
#10663=VECTOR('',#35520,1.);
#10664=VECTOR('',#35523,1.);
#10665=VECTOR('',#35524,1.);
#10666=VECTOR('',#35531,1.);
#10667=VECTOR('',#35532,1.);
#10668=VECTOR('',#35535,1.);
#10669=VECTOR('',#35536,1.);
#10670=VECTOR('',#35539,1.);
#10671=VECTOR('',#35544,0.925000000000001);
#10672=VECTOR('',#35551,0.875);
#10673=VECTOR('',#35554,1.);
#10674=VECTOR('',#35559,0.925000000000001);
#10675=VECTOR('',#35562,0.925000000000001);
#10676=VECTOR('',#35569,0.875);
#10677=VECTOR('',#35574,0.925000000000001);
#10678=VECTOR('',#35577,1.);
#10679=VECTOR('',#35582,0.925000000000001);
#10680=VECTOR('',#35589,0.875);
#10681=VECTOR('',#35592,0.925000000000001);
#10682=VECTOR('',#35595,0.925000000000001);
#10683=VECTOR('',#35602,0.875);
#10684=VECTOR('',#35605,0.925000000000001);
#10685=VECTOR('',#35608,0.949999999999999);
#10686=VECTOR('',#35613,0.899999999999999);
#10687=VECTOR('',#35618,0.949999999999999);
#10688=VECTOR('',#35623,0.899999999999999);
#10689=VECTOR('',#35628,1.);
#10690=VECTOR('',#35629,1.);
#10691=VECTOR('',#35630,1.);
#10692=VECTOR('',#35633,1.);
#10693=VECTOR('',#35640,1.);
#10694=VECTOR('',#35641,1.);
#10695=VECTOR('',#35642,1.);
#10696=VECTOR('',#35645,1.);
#10697=VECTOR('',#35652,1.);
#10698=VECTOR('',#35653,1.);
#10699=VECTOR('',#35656,1.);
#10700=VECTOR('',#35657,1.);
#10701=VECTOR('',#35660,1.);
#10702=VECTOR('',#35663,1.);
#10703=VECTOR('',#35670,1.);
#10704=VECTOR('',#35671,1.);
#10705=VECTOR('',#35674,1.);
#10706=VECTOR('',#35679,1.);
#10707=VECTOR('',#35680,1.);
#10708=VECTOR('',#35683,1.);
#10709=VECTOR('',#35688,1.);
#10710=VECTOR('',#35689,1.);
#10711=VECTOR('',#35692,0.949999999999999);
#10712=VECTOR('',#35695,0.949999999999999);
#10713=VECTOR('',#35698,1.);
#10714=VECTOR('',#35701,1.);
#10715=VECTOR('',#35702,1.);
#10716=VECTOR('',#35705,1.);
#10717=VECTOR('',#35708,1.);
#10718=VECTOR('',#35709,1.);
#10719=VECTOR('',#35712,1.);
#10720=VECTOR('',#35715,1.);
#10721=VECTOR('',#35718,1.);
#10722=VECTOR('',#35721,1.);
#10723=VECTOR('',#35726,1.);
#10724=VECTOR('',#35727,1.);
#10725=VECTOR('',#35730,1.);
#10726=VECTOR('',#35735,1.);
#10727=VECTOR('',#35738,1.);
#10728=VECTOR('',#35739,1.);
#10729=VECTOR('',#35742,1.);
#12885=VERTEX_POINT('',#50004);
#12886=VERTEX_POINT('',#50005);
#12887=VERTEX_POINT('',#50007);
#12888=VERTEX_POINT('',#50009);
#12889=VERTEX_POINT('',#50013);
#12890=VERTEX_POINT('',#50015);
#12891=VERTEX_POINT('',#50019);
#12892=VERTEX_POINT('',#50021);
#12893=VERTEX_POINT('',#50025);
#12894=VERTEX_POINT('',#50026);
#12895=VERTEX_POINT('',#50028);
#12896=VERTEX_POINT('',#50030);
#12897=VERTEX_POINT('',#50034);
#12898=VERTEX_POINT('',#50036);
#12899=VERTEX_POINT('',#50040);
#12900=VERTEX_POINT('',#50042);
#12901=VERTEX_POINT('',#50046);
#12902=VERTEX_POINT('',#50047);
#12903=VERTEX_POINT('',#50049);
#12904=VERTEX_POINT('',#50051);
#12905=VERTEX_POINT('',#50053);
#12906=VERTEX_POINT('',#50057);
#12907=VERTEX_POINT('',#50059);
#12908=VERTEX_POINT('',#50061);
#12909=VERTEX_POINT('',#50063);
#12910=VERTEX_POINT('',#50065);
#12911=VERTEX_POINT('',#50067);
#12912=VERTEX_POINT('',#50071);
#12913=VERTEX_POINT('',#50075);
#12914=VERTEX_POINT('',#50077);
#12915=VERTEX_POINT('',#50079);
#12916=VERTEX_POINT('',#50083);
#12917=VERTEX_POINT('',#50087);
#12918=VERTEX_POINT('',#50089);
#12919=VERTEX_POINT('',#50091);
#12920=VERTEX_POINT('',#50096);
#12921=VERTEX_POINT('',#50098);
#12922=VERTEX_POINT('',#50100);
#12923=VERTEX_POINT('',#50102);
#12924=VERTEX_POINT('',#50106);
#12925=VERTEX_POINT('',#50108);
#12926=VERTEX_POINT('',#50110);
#12927=VERTEX_POINT('',#50112);
#12928=VERTEX_POINT('',#50116);
#12929=VERTEX_POINT('',#50118);
#12930=VERTEX_POINT('',#50120);
#12931=VERTEX_POINT('',#50124);
#12932=VERTEX_POINT('',#50126);
#12933=VERTEX_POINT('',#50130);
#12934=VERTEX_POINT('',#50132);
#12935=VERTEX_POINT('',#50134);
#12936=VERTEX_POINT('',#50138);
#12937=VERTEX_POINT('',#50142);
#12938=VERTEX_POINT('',#50144);
#12939=VERTEX_POINT('',#50148);
#12940=VERTEX_POINT('',#50149);
#12941=VERTEX_POINT('',#50151);
#12942=VERTEX_POINT('',#50153);
#12943=VERTEX_POINT('',#50155);
#12944=VERTEX_POINT('',#50159);
#12945=VERTEX_POINT('',#50161);
#12946=VERTEX_POINT('',#50163);
#12947=VERTEX_POINT('',#50165);
#12948=VERTEX_POINT('',#50167);
#12949=VERTEX_POINT('',#50169);
#12950=VERTEX_POINT('',#50173);
#12951=VERTEX_POINT('',#50177);
#12952=VERTEX_POINT('',#50179);
#12953=VERTEX_POINT('',#50181);
#12954=VERTEX_POINT('',#50186);
#12955=VERTEX_POINT('',#50188);
#12956=VERTEX_POINT('',#50192);
#12957=VERTEX_POINT('',#50197);
#12958=VERTEX_POINT('',#50199);
#12959=VERTEX_POINT('',#50203);
#12960=VERTEX_POINT('',#50207);
#12961=VERTEX_POINT('',#50211);
#12962=VERTEX_POINT('',#50213);
#12963=VERTEX_POINT('',#50215);
#12964=VERTEX_POINT('',#50217);
#12965=VERTEX_POINT('',#50221);
#12966=VERTEX_POINT('',#50223);
#12967=VERTEX_POINT('',#50225);
#12968=VERTEX_POINT('',#50227);
#12969=VERTEX_POINT('',#50231);
#12970=VERTEX_POINT('',#50233);
#12971=VERTEX_POINT('',#50235);
#12972=VERTEX_POINT('',#50239);
#12973=VERTEX_POINT('',#50241);
#12974=VERTEX_POINT('',#50245);
#12975=VERTEX_POINT('',#50247);
#12976=VERTEX_POINT('',#50249);
#12977=VERTEX_POINT('',#50253);
#12978=VERTEX_POINT('',#50255);
#12979=VERTEX_POINT('',#50259);
#12980=VERTEX_POINT('',#50260);
#12981=VERTEX_POINT('',#50262);
#12982=VERTEX_POINT('',#50264);
#12983=VERTEX_POINT('',#50268);
#12984=VERTEX_POINT('',#50269);
#12985=VERTEX_POINT('',#50274);
#12986=VERTEX_POINT('',#50275);
#12987=VERTEX_POINT('',#50280);
#12988=VERTEX_POINT('',#50281);
#12989=VERTEX_POINT('',#50286);
#12990=VERTEX_POINT('',#50287);
#12991=VERTEX_POINT('',#50292);
#12992=VERTEX_POINT('',#50293);
#12993=VERTEX_POINT('',#50298);
#12994=VERTEX_POINT('',#50299);
#12995=VERTEX_POINT('',#50307);
#12996=VERTEX_POINT('',#50309);
#12997=VERTEX_POINT('',#50313);
#12998=VERTEX_POINT('',#50317);
#12999=VERTEX_POINT('',#50321);
#13000=VERTEX_POINT('',#50325);
#13001=VERTEX_POINT('',#50327);
#13002=VERTEX_POINT('',#50330);
#13003=VERTEX_POINT('',#50334);
#13004=VERTEX_POINT('',#50338);
#13005=VERTEX_POINT('',#50340);
#13006=VERTEX_POINT('',#50346);
#13007=VERTEX_POINT('',#50348);
#13008=VERTEX_POINT('',#50351);
#13009=VERTEX_POINT('',#50353);
#13010=VERTEX_POINT('',#50360);
#13011=VERTEX_POINT('',#50362);
#13012=VERTEX_POINT('',#50364);
#13013=VERTEX_POINT('',#50372);
#13014=VERTEX_POINT('',#50374);
#13015=VERTEX_POINT('',#50377);
#13016=VERTEX_POINT('',#50381);
#13017=VERTEX_POINT('',#50387);
#13018=VERTEX_POINT('',#50389);
#13019=VERTEX_POINT('',#50393);
#13020=VERTEX_POINT('',#50398);
#13021=VERTEX_POINT('',#50403);
#13022=VERTEX_POINT('',#50407);
#13023=VERTEX_POINT('',#50411);
#13024=VERTEX_POINT('',#50416);
#13025=VERTEX_POINT('',#50419);
#13026=VERTEX_POINT('',#50423);
#13027=VERTEX_POINT('',#50429);
#13028=VERTEX_POINT('',#50433);
#13029=VERTEX_POINT('',#50439);
#13030=VERTEX_POINT('',#50443);
#13031=VERTEX_POINT('',#50447);
#13032=VERTEX_POINT('',#50451);
#13033=VERTEX_POINT('',#50455);
#13034=VERTEX_POINT('',#50457);
#13035=VERTEX_POINT('',#50461);
#13036=VERTEX_POINT('',#50462);
#13037=VERTEX_POINT('',#50467);
#13038=VERTEX_POINT('',#50468);
#13039=VERTEX_POINT('',#50473);
#13040=VERTEX_POINT('',#50474);
#13041=VERTEX_POINT('',#50482);
#13042=VERTEX_POINT('',#50484);
#13043=VERTEX_POINT('',#50486);
#13044=VERTEX_POINT('',#50488);
#13045=VERTEX_POINT('',#50490);
#13046=VERTEX_POINT('',#50493);
#13047=VERTEX_POINT('',#50495);
#13048=VERTEX_POINT('',#50498);
#13049=VERTEX_POINT('',#50502);
#13050=VERTEX_POINT('',#50506);
#13051=VERTEX_POINT('',#50510);
#13052=VERTEX_POINT('',#50514);
#13053=VERTEX_POINT('',#50524);
#13054=VERTEX_POINT('',#50539);
#13055=VERTEX_POINT('',#50543);
#13056=VERTEX_POINT('',#50547);
#16406=EDGE_CURVE('',#12885,#12886,#8008,.F.);
#16407=EDGE_CURVE('',#12886,#12887,#8009,.T.);
#16408=EDGE_CURVE('',#12887,#12888,#8010,.F.);
#16409=EDGE_CURVE('',#12888,#12885,#8011,.T.);
#16410=EDGE_CURVE('',#12889,#12886,#8012,.T.);
#16411=EDGE_CURVE('',#12890,#12889,#8013,.T.);
#16412=EDGE_CURVE('',#12887,#12890,#8014,.T.);
#16413=EDGE_CURVE('',#12891,#12890,#8015,.F.);
#16414=EDGE_CURVE('',#12889,#12892,#8016,.F.);
#16415=EDGE_CURVE('',#12892,#12891,#8017,.T.);
#16416=EDGE_CURVE('',#12893,#12894,#8018,.F.);
#16417=EDGE_CURVE('',#12894,#12895,#8019,.T.);
#16418=EDGE_CURVE('',#12895,#12896,#8020,.F.);
#16419=EDGE_CURVE('',#12896,#12893,#8021,.T.);
#16420=EDGE_CURVE('',#12897,#12894,#8022,.T.);
#16421=EDGE_CURVE('',#12898,#12897,#8023,.T.);
#16422=EDGE_CURVE('',#12895,#12898,#8024,.T.);
#16423=EDGE_CURVE('',#12899,#12898,#8025,.F.);
#16424=EDGE_CURVE('',#12897,#12900,#8026,.F.);
#16425=EDGE_CURVE('',#12900,#12899,#8027,.T.);
#16426=EDGE_CURVE('',#12901,#12902,#8028,.T.);
#16427=EDGE_CURVE('',#12902,#12903,#8029,.T.);
#16428=EDGE_CURVE('',#12903,#12904,#8030,.F.);
#16429=EDGE_CURVE('',#12904,#12905,#8031,.T.);
#16430=EDGE_CURVE('',#12905,#12901,#8032,.T.);
#16431=EDGE_CURVE('',#12906,#12904,#8033,.T.);
#16432=EDGE_CURVE('',#12906,#12907,#8034,.T.);
#16433=EDGE_CURVE('',#12907,#12908,#8035,.T.);
#16434=EDGE_CURVE('',#12908,#12909,#8036,.T.);
#16435=EDGE_CURVE('',#12910,#12909,#8037,.T.);
#16436=EDGE_CURVE('',#12911,#12910,#8038,.T.);
#16437=EDGE_CURVE('',#12911,#12905,#8039,.T.);
#16438=EDGE_CURVE('',#12912,#12906,#8040,.T.);
#16439=EDGE_CURVE('',#12907,#12912,#8041,.F.);
#16440=EDGE_CURVE('',#12913,#12910,#8042,.T.);
#16441=EDGE_CURVE('',#12913,#12914,#8043,.T.);
#16442=EDGE_CURVE('',#12914,#12915,#8044,.T.);
#16443=EDGE_CURVE('',#12915,#12911,#8045,.T.);
#16444=EDGE_CURVE('',#12909,#12916,#8046,.T.);
#16445=EDGE_CURVE('',#12908,#12916,#8047,.T.);
#16446=EDGE_CURVE('',#12917,#12900,#8048,.T.);
#16447=EDGE_CURVE('',#12918,#12917,#8049,.F.);
#16448=EDGE_CURVE('',#12918,#12919,#8050,.T.);
#16449=EDGE_CURVE('',#12919,#12914,#8051,.T.);
#16450=EDGE_CURVE('',#12899,#12913,#8052,.T.);
#16451=EDGE_CURVE('',#12920,#12907,#8053,.T.);
#16452=EDGE_CURVE('',#12921,#12920,#8054,.T.);
#16453=EDGE_CURVE('',#12922,#12921,#8055,.T.);
#16454=EDGE_CURVE('',#12923,#12922,#8056,.T.);
#16455=EDGE_CURVE('',#12908,#12923,#8057,.T.);
#16456=EDGE_CURVE('',#12924,#12921,#8058,.T.);
#16457=EDGE_CURVE('',#12920,#12925,#8059,.T.);
#16458=EDGE_CURVE('',#12925,#12926,#8060,.T.);
#16459=EDGE_CURVE('',#12926,#12927,#8061,.T.);
#16460=EDGE_CURVE('',#12927,#12924,#8062,.T.);
#16461=EDGE_CURVE('',#12928,#12924,#8063,.T.);
#16462=EDGE_CURVE('',#12928,#12929,#8064,.T.);
#16463=EDGE_CURVE('',#12930,#12929,#8065,.T.);
#16464=EDGE_CURVE('',#12922,#12930,#8066,.T.);
#16465=EDGE_CURVE('',#12927,#12931,#8067,.T.);
#16466=EDGE_CURVE('',#12931,#12932,#8068,.F.);
#16467=EDGE_CURVE('',#12932,#12928,#8069,.T.);
#16468=EDGE_CURVE('',#12933,#12923,#8070,.T.);
#16469=EDGE_CURVE('',#12930,#12934,#8071,.T.);
#16470=EDGE_CURVE('',#12934,#12935,#8072,.T.);
#16471=EDGE_CURVE('',#12935,#12933,#8073,.T.);
#16472=EDGE_CURVE('',#12936,#12933,#8074,.T.);
#16473=EDGE_CURVE('',#12936,#12916,#8075,.T.);
#16474=EDGE_CURVE('',#12935,#12937,#8076,.T.);
#16475=EDGE_CURVE('',#12937,#12938,#8077,.F.);
#16476=EDGE_CURVE('',#12938,#12936,#8078,.T.);
#16477=EDGE_CURVE('',#12939,#12940,#8079,.T.);
#16478=EDGE_CURVE('',#12941,#12940,#8080,.T.);
#16479=EDGE_CURVE('',#12941,#12942,#8081,.T.);
#16480=EDGE_CURVE('',#12942,#12943,#8082,.T.);
#16481=EDGE_CURVE('',#12943,#12939,#8083,.T.);
#16482=EDGE_CURVE('',#12940,#12944,#8084,.T.);
#16483=EDGE_CURVE('',#12939,#12945,#8085,.T.);
#16484=EDGE_CURVE('',#12946,#12945,#8086,.T.);
#16485=EDGE_CURVE('',#12947,#12946,#8087,.T.);
#16486=EDGE_CURVE('',#12947,#12948,#8088,.T.);
#16487=EDGE_CURVE('',#12948,#12949,#8089,.T.);
#16488=EDGE_CURVE('',#12949,#12944,#8090,.T.);
#16489=EDGE_CURVE('',#12943,#12950,#8091,.T.);
#16490=EDGE_CURVE('',#12945,#12950,#8092,.T.);
#16491=EDGE_CURVE('',#12951,#12888,#8093,.T.);
#16492=EDGE_CURVE('',#12952,#12951,#8094,.F.);
#16493=EDGE_CURVE('',#12952,#12953,#8095,.T.);
#16494=EDGE_CURVE('',#12953,#12942,#8096,.T.);
#16495=EDGE_CURVE('',#12885,#12941,#8097,.T.);
#16496=EDGE_CURVE('',#12954,#12953,#8098,.T.);
#16497=EDGE_CURVE('',#12955,#12954,#8099,.T.);
#16498=EDGE_CURVE('',#12950,#12955,#8100,.T.);
#16499=EDGE_CURVE('',#12955,#12956,#8101,.T.);
#16500=EDGE_CURVE('',#12956,#12946,#8102,.F.);
#16501=EDGE_CURVE('',#12956,#12892,#8103,.T.);
#16502=EDGE_CURVE('',#12954,#12957,#8104,.T.);
#16503=EDGE_CURVE('',#12957,#12958,#8105,.T.);
#16504=EDGE_CURVE('',#12891,#12958,#8106,.T.);
#16505=EDGE_CURVE('',#12959,#12947,#8107,.T.);
#16506=EDGE_CURVE('',#12948,#12959,#8108,.F.);
#16507=EDGE_CURVE('',#12944,#12960,#8109,.T.);
#16508=EDGE_CURVE('',#12949,#12960,#8110,.T.);
#16509=EDGE_CURVE('',#12961,#12948,#8111,.T.);
#16510=EDGE_CURVE('',#12962,#12961,#8112,.T.);
#16511=EDGE_CURVE('',#12963,#12962,#8113,.T.);
#16512=EDGE_CURVE('',#12964,#12963,#8114,.T.);
#16513=EDGE_CURVE('',#12949,#12964,#8115,.T.);
#16514=EDGE_CURVE('',#12965,#12964,#8116,.T.);
#16515=EDGE_CURVE('',#12963,#12966,#8117,.T.);
#16516=EDGE_CURVE('',#12966,#12967,#8118,.T.);
#16517=EDGE_CURVE('',#12967,#12968,#8119,.T.);
#16518=EDGE_CURVE('',#12968,#12965,#8120,.T.);
#16519=EDGE_CURVE('',#12966,#12969,#8121,.T.);
#16520=EDGE_CURVE('',#12969,#12970,#8122,.T.);
#16521=EDGE_CURVE('',#12970,#12971,#8123,.F.);
#16522=EDGE_CURVE('',#12971,#12967,#8124,.T.);
#16523=EDGE_CURVE('',#12972,#12962,#8125,.T.);
#16524=EDGE_CURVE('',#12973,#12972,#8126,.T.);
#16525=EDGE_CURVE('',#12973,#12969,#8127,.T.);
#16526=EDGE_CURVE('',#12961,#12974,#8128,.T.);
#16527=EDGE_CURVE('',#12974,#12975,#8129,.T.);
#16528=EDGE_CURVE('',#12975,#12976,#8130,.T.);
#16529=EDGE_CURVE('',#12976,#12972,#8131,.T.);
#16530=EDGE_CURVE('',#12976,#12977,#8132,.T.);
#16531=EDGE_CURVE('',#12977,#12978,#8133,.F.);
#16532=EDGE_CURVE('',#12978,#12973,#8134,.T.);
#16533=EDGE_CURVE('',#12979,#12980,#8135,.T.);
#16534=EDGE_CURVE('',#12980,#12981,#2479,.T.);
#16535=EDGE_CURVE('',#12981,#12982,#8136,.T.);
#16536=EDGE_CURVE('',#12982,#12979,#2480,.T.);
#16537=EDGE_CURVE('',#12983,#12984,#8137,.T.);
#16538=EDGE_CURVE('',#12984,#12980,#8138,.T.);
#16539=EDGE_CURVE('',#12979,#12983,#8139,.T.);
#16540=EDGE_CURVE('',#12985,#12986,#8140,.T.);
#16541=EDGE_CURVE('',#12986,#12984,#2481,.T.);
#16542=EDGE_CURVE('',#12983,#12985,#2482,.T.);
#16543=EDGE_CURVE('',#12987,#12988,#8141,.T.);
#16544=EDGE_CURVE('',#12988,#12986,#8142,.T.);
#16545=EDGE_CURVE('',#12985,#12987,#8143,.T.);
#16546=EDGE_CURVE('',#12989,#12990,#8144,.T.);
#16547=EDGE_CURVE('',#12990,#12988,#2483,.T.);
#16548=EDGE_CURVE('',#12987,#12989,#2484,.T.);
#16549=EDGE_CURVE('',#12991,#12992,#8145,.T.);
#16550=EDGE_CURVE('',#12992,#12990,#8146,.T.);
#16551=EDGE_CURVE('',#12989,#12991,#8147,.T.);
#16552=EDGE_CURVE('',#12993,#12994,#8148,.T.);
#16553=EDGE_CURVE('',#12994,#12992,#2485,.T.);
#16554=EDGE_CURVE('',#12991,#12993,#2486,.T.);
#16555=EDGE_CURVE('',#12981,#12994,#8149,.T.);
#16556=EDGE_CURVE('',#12993,#12982,#8150,.T.);
#16557=EDGE_CURVE('',#12995,#12992,#8151,.T.);
#16558=EDGE_CURVE('',#12996,#12995,#8152,.T.);
#16559=EDGE_CURVE('',#12990,#12996,#8153,.T.);
#16560=EDGE_CURVE('',#12994,#12997,#8154,.T.);
#16561=EDGE_CURVE('',#12995,#12997,#2487,.T.);
#16562=EDGE_CURVE('',#12998,#12981,#8155,.T.);
#16563=EDGE_CURVE('',#12997,#12998,#8156,.T.);
#16564=EDGE_CURVE('',#12980,#12999,#8157,.T.);
#16565=EDGE_CURVE('',#12998,#12999,#2488,.T.);
#16566=EDGE_CURVE('',#13000,#13000,#2489,.T.);
#16567=EDGE_CURVE('',#13001,#13001,#2490,.T.);
#16568=EDGE_CURVE('',#13002,#12975,#8158,.T.);
#16569=EDGE_CURVE('',#12977,#13002,#8159,.T.);
#16570=EDGE_CURVE('',#13003,#12971,#8160,.T.);
#16571=EDGE_CURVE('',#12968,#13003,#8161,.T.);
#16572=EDGE_CURVE('',#12974,#13004,#8162,.T.);
#16573=EDGE_CURVE('',#13004,#13005,#8163,.T.);
#16574=EDGE_CURVE('',#13005,#13002,#8164,.F.);
#16575=EDGE_CURVE('',#12959,#13004,#8165,.T.);
#16576=EDGE_CURVE('',#13006,#12960,#8166,.T.);
#16577=EDGE_CURVE('',#13007,#13006,#8167,.T.);
#16578=EDGE_CURVE('',#13005,#13007,#8168,.T.);
#16579=EDGE_CURVE('',#13008,#13008,#2491,.T.);
#16580=EDGE_CURVE('',#13009,#13009,#2492,.T.);
#16581=EDGE_CURVE('',#13003,#13007,#8169,.F.);
#16582=EDGE_CURVE('',#13006,#12965,#8170,.T.);
#16583=EDGE_CURVE('',#12925,#13010,#8171,.T.);
#16584=EDGE_CURVE('',#13010,#13011,#8172,.T.);
#16585=EDGE_CURVE('',#13011,#13012,#8173,.F.);
#16586=EDGE_CURVE('',#13012,#12926,#8174,.T.);
#16587=EDGE_CURVE('',#12912,#13010,#8175,.T.);
#16588=EDGE_CURVE('',#12903,#12896,#8176,.T.);
#16589=EDGE_CURVE('',#13011,#12938,#8177,.T.);
#16590=EDGE_CURVE('',#13013,#13013,#2493,.T.);
#16591=EDGE_CURVE('',#13014,#13014,#2494,.T.);
#16592=EDGE_CURVE('',#13015,#12934,#8178,.T.);
#16593=EDGE_CURVE('',#12937,#13015,#8179,.T.);
#16594=EDGE_CURVE('',#12929,#13016,#8180,.T.);
#16595=EDGE_CURVE('',#13016,#13015,#8181,.F.);
#16596=EDGE_CURVE('',#12931,#13012,#8182,.T.);
#16597=EDGE_CURVE('',#13017,#13017,#2495,.T.);
#16598=EDGE_CURVE('',#13017,#13018,#8183,.T.);
#16599=EDGE_CURVE('',#13018,#13018,#2496,.T.);
#16600=EDGE_CURVE('',#13019,#13019,#2497,.T.);
#16601=EDGE_CURVE('',#13019,#13018,#8184,.T.);
#16602=EDGE_CURVE('',#13016,#12932,#8185,.T.);
#16603=EDGE_CURVE('',#13020,#13020,#2498,.T.);
#16604=EDGE_CURVE('',#13013,#13019,#8186,.T.);
#16605=EDGE_CURVE('',#13008,#13021,#8187,.T.);
#16606=EDGE_CURVE('',#13021,#13021,#2499,.T.);
#16607=EDGE_CURVE('',#13022,#13022,#2500,.T.);
#16608=EDGE_CURVE('',#13022,#13021,#8188,.T.);
#16609=EDGE_CURVE('',#13023,#13023,#2501,.T.);
#16610=EDGE_CURVE('',#13023,#13022,#8189,.T.);
#16611=EDGE_CURVE('',#12970,#12978,#8190,.T.);
#16612=EDGE_CURVE('',#13024,#13024,#2502,.T.);
#16613=EDGE_CURVE('',#13020,#13025,#8191,.T.);
#16614=EDGE_CURVE('',#13025,#13025,#2503,.T.);
#16615=EDGE_CURVE('',#13026,#13026,#2504,.T.);
#16616=EDGE_CURVE('',#13026,#13025,#8192,.T.);
#16617=EDGE_CURVE('',#13014,#13026,#8193,.T.);
#16618=EDGE_CURVE('',#13009,#13027,#8194,.T.);
#16619=EDGE_CURVE('',#13027,#13027,#2505,.T.);
#16620=EDGE_CURVE('',#13028,#13028,#2506,.T.);
#16621=EDGE_CURVE('',#13028,#13027,#8195,.T.);
#16622=EDGE_CURVE('',#13024,#13028,#8196,.T.);
#16623=EDGE_CURVE('',#13000,#13029,#8197,.T.);
#16624=EDGE_CURVE('',#13029,#13029,#2507,.T.);
#16625=EDGE_CURVE('',#13029,#13030,#8198,.T.);
#16626=EDGE_CURVE('',#13030,#13030,#2508,.T.);
#16627=EDGE_CURVE('',#13001,#13031,#8199,.T.);
#16628=EDGE_CURVE('',#13031,#13031,#2509,.T.);
#16629=EDGE_CURVE('',#13031,#13032,#8200,.T.);
#16630=EDGE_CURVE('',#13032,#13032,#2510,.T.);
#16631=EDGE_CURVE('',#12917,#13033,#8201,.T.);
#16632=EDGE_CURVE('',#13033,#13034,#8202,.T.);
#16633=EDGE_CURVE('',#13034,#12918,#8203,.T.);
#16634=EDGE_CURVE('',#13035,#13036,#8204,.T.);
#16635=EDGE_CURVE('',#13036,#13034,#2511,.T.);
#16636=EDGE_CURVE('',#13033,#13035,#2512,.T.);
#16637=EDGE_CURVE('',#13037,#13038,#8205,.T.);
#16638=EDGE_CURVE('',#13038,#13036,#8206,.T.);
#16639=EDGE_CURVE('',#13035,#13037,#8207,.T.);
#16640=EDGE_CURVE('',#13039,#13040,#8208,.T.);
#16641=EDGE_CURVE('',#13040,#13038,#2513,.T.);
#16642=EDGE_CURVE('',#13037,#13039,#2514,.T.);
#16643=EDGE_CURVE('',#12957,#13040,#8209,.T.);
#16644=EDGE_CURVE('',#13039,#12958,#8210,.T.);
#16645=EDGE_CURVE('',#12893,#13041,#8211,.T.);
#16646=EDGE_CURVE('',#13042,#13041,#8212,.T.);
#16647=EDGE_CURVE('',#13043,#13042,#2515,.T.);
#16648=EDGE_CURVE('',#13044,#13043,#8213,.T.);
#16649=EDGE_CURVE('',#13045,#13044,#2516,.T.);
#16650=EDGE_CURVE('',#12951,#13045,#8214,.T.);
#16651=EDGE_CURVE('',#13046,#13046,#2517,.T.);
#16652=EDGE_CURVE('',#13047,#13047,#2518,.T.);
#16653=EDGE_CURVE('',#13045,#13048,#8215,.T.);
#16654=EDGE_CURVE('',#13048,#12952,#8216,.T.);
#16655=EDGE_CURVE('',#13044,#13049,#8217,.T.);
#16656=EDGE_CURVE('',#13049,#13048,#2519,.T.);
#16657=EDGE_CURVE('',#13043,#13050,#8218,.T.);
#16658=EDGE_CURVE('',#13050,#13049,#8219,.T.);
#16659=EDGE_CURVE('',#13042,#13051,#8220,.T.);
#16660=EDGE_CURVE('',#13051,#13050,#2520,.T.);
#16661=EDGE_CURVE('',#13052,#13041,#8221,.T.);
#16662=EDGE_CURVE('',#13052,#13051,#8222,.T.);
#16663=EDGE_CURVE('',#13047,#13032,#8223,.T.);
#16664=EDGE_CURVE('',#13046,#13030,#8224,.T.);
#16665=EDGE_CURVE('',#12901,#12915,#8225,.T.);
#16666=EDGE_CURVE('',#13053,#12919,#8226,.T.);
#16667=EDGE_CURVE('',#12902,#13053,#8227,.T.);
#16668=EDGE_CURVE('',#13053,#13052,#8228,.T.);
#16669=EDGE_CURVE('',#13036,#12998,#8229,.T.);
#16670=EDGE_CURVE('',#12999,#13034,#8230,.T.);
#16671=EDGE_CURVE('',#13038,#12997,#8231,.T.);
#16672=EDGE_CURVE('',#13040,#12995,#8232,.T.);
#16673=EDGE_CURVE('',#13048,#12996,#8233,.T.);
#16674=EDGE_CURVE('',#13049,#13054,#8234,.T.);
#16675=EDGE_CURVE('',#13054,#12996,#2521,.T.);
#16676=EDGE_CURVE('',#13050,#13055,#8235,.T.);
#16677=EDGE_CURVE('',#13055,#13054,#8236,.T.);
#16678=EDGE_CURVE('',#13051,#13056,#8237,.T.);
#16679=EDGE_CURVE('',#13056,#13055,#2522,.T.);
#16680=EDGE_CURVE('',#12999,#13056,#8238,.T.);
#16681=EDGE_CURVE('',#13054,#12988,#8239,.T.);
#16682=EDGE_CURVE('',#12986,#13055,#8240,.T.);
#16683=EDGE_CURVE('',#13056,#12984,#8241,.T.);
#23045=ORIENTED_EDGE('',*,*,#16406,.T.);
#23046=ORIENTED_EDGE('',*,*,#16407,.T.);
#23047=ORIENTED_EDGE('',*,*,#16408,.T.);
#23048=ORIENTED_EDGE('',*,*,#16409,.T.);
#23049=ORIENTED_EDGE('',*,*,#16407,.F.);
#23050=ORIENTED_EDGE('',*,*,#16410,.F.);
#23051=ORIENTED_EDGE('',*,*,#16411,.F.);
#23052=ORIENTED_EDGE('',*,*,#16412,.F.);
#23053=ORIENTED_EDGE('',*,*,#16413,.T.);
#23054=ORIENTED_EDGE('',*,*,#16411,.T.);
#23055=ORIENTED_EDGE('',*,*,#16414,.T.);
#23056=ORIENTED_EDGE('',*,*,#16415,.T.);
#23057=ORIENTED_EDGE('',*,*,#16416,.T.);
#23058=ORIENTED_EDGE('',*,*,#16417,.T.);
#23059=ORIENTED_EDGE('',*,*,#16418,.T.);
#23060=ORIENTED_EDGE('',*,*,#16419,.T.);
#23061=ORIENTED_EDGE('',*,*,#16417,.F.);
#23062=ORIENTED_EDGE('',*,*,#16420,.F.);
#23063=ORIENTED_EDGE('',*,*,#16421,.F.);
#23064=ORIENTED_EDGE('',*,*,#16422,.F.);
#23065=ORIENTED_EDGE('',*,*,#16423,.T.);
#23066=ORIENTED_EDGE('',*,*,#16421,.T.);
#23067=ORIENTED_EDGE('',*,*,#16424,.T.);
#23068=ORIENTED_EDGE('',*,*,#16425,.T.);
#23069=ORIENTED_EDGE('',*,*,#16426,.T.);
#23070=ORIENTED_EDGE('',*,*,#16427,.T.);
#23071=ORIENTED_EDGE('',*,*,#16428,.T.);
#23072=ORIENTED_EDGE('',*,*,#16429,.T.);
#23073=ORIENTED_EDGE('',*,*,#16430,.T.);
#23074=ORIENTED_EDGE('',*,*,#16429,.F.);
#23075=ORIENTED_EDGE('',*,*,#16431,.F.);
#23076=ORIENTED_EDGE('',*,*,#16432,.T.);
#23077=ORIENTED_EDGE('',*,*,#16433,.T.);
#23078=ORIENTED_EDGE('',*,*,#16434,.T.);
#23079=ORIENTED_EDGE('',*,*,#16435,.F.);
#23080=ORIENTED_EDGE('',*,*,#16436,.F.);
#23081=ORIENTED_EDGE('',*,*,#16437,.T.);
#23082=ORIENTED_EDGE('',*,*,#16438,.F.);
#23083=ORIENTED_EDGE('',*,*,#16439,.F.);
#23084=ORIENTED_EDGE('',*,*,#16432,.F.);
#23085=ORIENTED_EDGE('',*,*,#16436,.T.);
#23086=ORIENTED_EDGE('',*,*,#16440,.F.);
#23087=ORIENTED_EDGE('',*,*,#16441,.T.);
#23088=ORIENTED_EDGE('',*,*,#16442,.T.);
#23089=ORIENTED_EDGE('',*,*,#16443,.T.);
#23090=ORIENTED_EDGE('',*,*,#16444,.F.);
#23091=ORIENTED_EDGE('',*,*,#16434,.F.);
#23092=ORIENTED_EDGE('',*,*,#16445,.T.);
#23093=ORIENTED_EDGE('',*,*,#16425,.F.);
#23094=ORIENTED_EDGE('',*,*,#16446,.F.);
#23095=ORIENTED_EDGE('',*,*,#16447,.F.);
#23096=ORIENTED_EDGE('',*,*,#16448,.T.);
#23097=ORIENTED_EDGE('',*,*,#16449,.T.);
#23098=ORIENTED_EDGE('',*,*,#16441,.F.);
#23099=ORIENTED_EDGE('',*,*,#16450,.F.);
#23100=ORIENTED_EDGE('',*,*,#16433,.F.);
#23101=ORIENTED_EDGE('',*,*,#16451,.F.);
#23102=ORIENTED_EDGE('',*,*,#16452,.F.);
#23103=ORIENTED_EDGE('',*,*,#16453,.F.);
#23104=ORIENTED_EDGE('',*,*,#16454,.F.);
#23105=ORIENTED_EDGE('',*,*,#16455,.F.);
#23106=ORIENTED_EDGE('',*,*,#16456,.T.);
#23107=ORIENTED_EDGE('',*,*,#16452,.T.);
#23108=ORIENTED_EDGE('',*,*,#16457,.T.);
#23109=ORIENTED_EDGE('',*,*,#16458,.T.);
#23110=ORIENTED_EDGE('',*,*,#16459,.T.);
#23111=ORIENTED_EDGE('',*,*,#16460,.T.);
#23112=ORIENTED_EDGE('',*,*,#16456,.F.);
#23113=ORIENTED_EDGE('',*,*,#16461,.F.);
#23114=ORIENTED_EDGE('',*,*,#16462,.T.);
#23115=ORIENTED_EDGE('',*,*,#16463,.F.);
#23116=ORIENTED_EDGE('',*,*,#16464,.F.);
#23117=ORIENTED_EDGE('',*,*,#16453,.T.);
#23118=ORIENTED_EDGE('',*,*,#16460,.F.);
#23119=ORIENTED_EDGE('',*,*,#16465,.T.);
#23120=ORIENTED_EDGE('',*,*,#16466,.T.);
#23121=ORIENTED_EDGE('',*,*,#16467,.T.);
#23122=ORIENTED_EDGE('',*,*,#16461,.T.);
#23123=ORIENTED_EDGE('',*,*,#16468,.T.);
#23124=ORIENTED_EDGE('',*,*,#16454,.T.);
#23125=ORIENTED_EDGE('',*,*,#16464,.T.);
#23126=ORIENTED_EDGE('',*,*,#16469,.T.);
#23127=ORIENTED_EDGE('',*,*,#16470,.T.);
#23128=ORIENTED_EDGE('',*,*,#16471,.T.);
#23129=ORIENTED_EDGE('',*,*,#16468,.F.);
#23130=ORIENTED_EDGE('',*,*,#16472,.F.);
#23131=ORIENTED_EDGE('',*,*,#16473,.T.);
#23132=ORIENTED_EDGE('',*,*,#16445,.F.);
#23133=ORIENTED_EDGE('',*,*,#16455,.T.);
#23134=ORIENTED_EDGE('',*,*,#16471,.F.);
#23135=ORIENTED_EDGE('',*,*,#16474,.T.);
#23136=ORIENTED_EDGE('',*,*,#16475,.T.);
#23137=ORIENTED_EDGE('',*,*,#16476,.T.);
#23138=ORIENTED_EDGE('',*,*,#16472,.T.);
#23139=ORIENTED_EDGE('',*,*,#16477,.T.);
#23140=ORIENTED_EDGE('',*,*,#16478,.F.);
#23141=ORIENTED_EDGE('',*,*,#16479,.T.);
#23142=ORIENTED_EDGE('',*,*,#16480,.T.);
#23143=ORIENTED_EDGE('',*,*,#16481,.T.);
#23144=ORIENTED_EDGE('',*,*,#16482,.F.);
#23145=ORIENTED_EDGE('',*,*,#16477,.F.);
#23146=ORIENTED_EDGE('',*,*,#16483,.T.);
#23147=ORIENTED_EDGE('',*,*,#16484,.F.);
#23148=ORIENTED_EDGE('',*,*,#16485,.F.);
#23149=ORIENTED_EDGE('',*,*,#16486,.T.);
#23150=ORIENTED_EDGE('',*,*,#16487,.T.);
#23151=ORIENTED_EDGE('',*,*,#16488,.T.);
#23152=ORIENTED_EDGE('',*,*,#16481,.F.);
#23153=ORIENTED_EDGE('',*,*,#16489,.T.);
#23154=ORIENTED_EDGE('',*,*,#16490,.F.);
#23155=ORIENTED_EDGE('',*,*,#16483,.F.);
#23156=ORIENTED_EDGE('',*,*,#16409,.F.);
#23157=ORIENTED_EDGE('',*,*,#16491,.F.);
#23158=ORIENTED_EDGE('',*,*,#16492,.F.);
#23159=ORIENTED_EDGE('',*,*,#16493,.T.);
#23160=ORIENTED_EDGE('',*,*,#16494,.T.);
#23161=ORIENTED_EDGE('',*,*,#16479,.F.);
#23162=ORIENTED_EDGE('',*,*,#16495,.F.);
#23163=ORIENTED_EDGE('',*,*,#16480,.F.);
#23164=ORIENTED_EDGE('',*,*,#16494,.F.);
#23165=ORIENTED_EDGE('',*,*,#16496,.F.);
#23166=ORIENTED_EDGE('',*,*,#16497,.F.);
#23167=ORIENTED_EDGE('',*,*,#16498,.F.);
#23168=ORIENTED_EDGE('',*,*,#16489,.F.);
#23169=ORIENTED_EDGE('',*,*,#16498,.T.);
#23170=ORIENTED_EDGE('',*,*,#16499,.T.);
#23171=ORIENTED_EDGE('',*,*,#16500,.T.);
#23172=ORIENTED_EDGE('',*,*,#16484,.T.);
#23173=ORIENTED_EDGE('',*,*,#16490,.T.);
#23174=ORIENTED_EDGE('',*,*,#16415,.F.);
#23175=ORIENTED_EDGE('',*,*,#16501,.F.);
#23176=ORIENTED_EDGE('',*,*,#16499,.F.);
#23177=ORIENTED_EDGE('',*,*,#16497,.T.);
#23178=ORIENTED_EDGE('',*,*,#16502,.T.);
#23179=ORIENTED_EDGE('',*,*,#16503,.T.);
#23180=ORIENTED_EDGE('',*,*,#16504,.F.);
#23181=ORIENTED_EDGE('',*,*,#16505,.F.);
#23182=ORIENTED_EDGE('',*,*,#16506,.F.);
#23183=ORIENTED_EDGE('',*,*,#16486,.F.);
#23184=ORIENTED_EDGE('',*,*,#16507,.F.);
#23185=ORIENTED_EDGE('',*,*,#16488,.F.);
#23186=ORIENTED_EDGE('',*,*,#16508,.T.);
#23187=ORIENTED_EDGE('',*,*,#16487,.F.);
#23188=ORIENTED_EDGE('',*,*,#16509,.F.);
#23189=ORIENTED_EDGE('',*,*,#16510,.F.);
#23190=ORIENTED_EDGE('',*,*,#16511,.F.);
#23191=ORIENTED_EDGE('',*,*,#16512,.F.);
#23192=ORIENTED_EDGE('',*,*,#16513,.F.);
#23193=ORIENTED_EDGE('',*,*,#16514,.T.);
#23194=ORIENTED_EDGE('',*,*,#16512,.T.);
#23195=ORIENTED_EDGE('',*,*,#16515,.T.);
#23196=ORIENTED_EDGE('',*,*,#16516,.T.);
#23197=ORIENTED_EDGE('',*,*,#16517,.T.);
#23198=ORIENTED_EDGE('',*,*,#16518,.T.);
#23199=ORIENTED_EDGE('',*,*,#16516,.F.);
#23200=ORIENTED_EDGE('',*,*,#16519,.T.);
#23201=ORIENTED_EDGE('',*,*,#16520,.T.);
#23202=ORIENTED_EDGE('',*,*,#16521,.T.);
#23203=ORIENTED_EDGE('',*,*,#16522,.T.);
#23204=ORIENTED_EDGE('',*,*,#16515,.F.);
#23205=ORIENTED_EDGE('',*,*,#16511,.T.);
#23206=ORIENTED_EDGE('',*,*,#16523,.F.);
#23207=ORIENTED_EDGE('',*,*,#16524,.F.);
#23208=ORIENTED_EDGE('',*,*,#16525,.T.);
#23209=ORIENTED_EDGE('',*,*,#16519,.F.);
#23210=ORIENTED_EDGE('',*,*,#16523,.T.);
#23211=ORIENTED_EDGE('',*,*,#16510,.T.);
#23212=ORIENTED_EDGE('',*,*,#16526,.T.);
#23213=ORIENTED_EDGE('',*,*,#16527,.T.);
#23214=ORIENTED_EDGE('',*,*,#16528,.T.);
#23215=ORIENTED_EDGE('',*,*,#16529,.T.);
#23216=ORIENTED_EDGE('',*,*,#16529,.F.);
#23217=ORIENTED_EDGE('',*,*,#16530,.T.);
#23218=ORIENTED_EDGE('',*,*,#16531,.T.);
#23219=ORIENTED_EDGE('',*,*,#16532,.T.);
#23220=ORIENTED_EDGE('',*,*,#16524,.T.);
#23221=ORIENTED_EDGE('',*,*,#16533,.T.);
#23222=ORIENTED_EDGE('',*,*,#16534,.T.);
#23223=ORIENTED_EDGE('',*,*,#16535,.T.);
#23224=ORIENTED_EDGE('',*,*,#16536,.T.);
#23225=ORIENTED_EDGE('',*,*,#16537,.T.);
#23226=ORIENTED_EDGE('',*,*,#16538,.T.);
#23227=ORIENTED_EDGE('',*,*,#16533,.F.);
#23228=ORIENTED_EDGE('',*,*,#16539,.T.);
#23229=ORIENTED_EDGE('',*,*,#16540,.T.);
#23230=ORIENTED_EDGE('',*,*,#16541,.T.);
#23231=ORIENTED_EDGE('',*,*,#16537,.F.);
#23232=ORIENTED_EDGE('',*,*,#16542,.T.);
#23233=ORIENTED_EDGE('',*,*,#16543,.T.);
#23234=ORIENTED_EDGE('',*,*,#16544,.T.);
#23235=ORIENTED_EDGE('',*,*,#16540,.F.);
#23236=ORIENTED_EDGE('',*,*,#16545,.T.);
#23237=ORIENTED_EDGE('',*,*,#16546,.T.);
#23238=ORIENTED_EDGE('',*,*,#16547,.T.);
#23239=ORIENTED_EDGE('',*,*,#16543,.F.);
#23240=ORIENTED_EDGE('',*,*,#16548,.T.);
#23241=ORIENTED_EDGE('',*,*,#16549,.T.);
#23242=ORIENTED_EDGE('',*,*,#16550,.T.);
#23243=ORIENTED_EDGE('',*,*,#16546,.F.);
#23244=ORIENTED_EDGE('',*,*,#16551,.T.);
#23245=ORIENTED_EDGE('',*,*,#16552,.T.);
#23246=ORIENTED_EDGE('',*,*,#16553,.T.);
#23247=ORIENTED_EDGE('',*,*,#16549,.F.);
#23248=ORIENTED_EDGE('',*,*,#16554,.T.);
#23249=ORIENTED_EDGE('',*,*,#16535,.F.);
#23250=ORIENTED_EDGE('',*,*,#16555,.T.);
#23251=ORIENTED_EDGE('',*,*,#16552,.F.);
#23252=ORIENTED_EDGE('',*,*,#16556,.T.);
#23253=ORIENTED_EDGE('',*,*,#16550,.F.);
#23254=ORIENTED_EDGE('',*,*,#16557,.F.);
#23255=ORIENTED_EDGE('',*,*,#16558,.F.);
#23256=ORIENTED_EDGE('',*,*,#16559,.F.);
#23257=ORIENTED_EDGE('',*,*,#16553,.F.);
#23258=ORIENTED_EDGE('',*,*,#16560,.T.);
#23259=ORIENTED_EDGE('',*,*,#16561,.F.);
#23260=ORIENTED_EDGE('',*,*,#16557,.T.);
#23261=ORIENTED_EDGE('',*,*,#16555,.F.);
#23262=ORIENTED_EDGE('',*,*,#16562,.F.);
#23263=ORIENTED_EDGE('',*,*,#16563,.F.);
#23264=ORIENTED_EDGE('',*,*,#16560,.F.);
#23265=ORIENTED_EDGE('',*,*,#16534,.F.);
#23266=ORIENTED_EDGE('',*,*,#16564,.T.);
#23267=ORIENTED_EDGE('',*,*,#16565,.F.);
#23268=ORIENTED_EDGE('',*,*,#16562,.T.);
#23269=ORIENTED_EDGE('',*,*,#16536,.F.);
#23270=ORIENTED_EDGE('',*,*,#16556,.F.);
#23271=ORIENTED_EDGE('',*,*,#16554,.F.);
#23272=ORIENTED_EDGE('',*,*,#16551,.F.);
#23273=ORIENTED_EDGE('',*,*,#16548,.F.);
#23274=ORIENTED_EDGE('',*,*,#16545,.F.);
#23275=ORIENTED_EDGE('',*,*,#16542,.F.);
#23276=ORIENTED_EDGE('',*,*,#16539,.F.);
#23277=ORIENTED_EDGE('',*,*,#16566,.F.);
#23278=ORIENTED_EDGE('',*,*,#16567,.F.);
#23279=ORIENTED_EDGE('',*,*,#16528,.F.);
#23280=ORIENTED_EDGE('',*,*,#16568,.F.);
#23281=ORIENTED_EDGE('',*,*,#16569,.F.);
#23282=ORIENTED_EDGE('',*,*,#16530,.F.);
#23283=ORIENTED_EDGE('',*,*,#16517,.F.);
#23284=ORIENTED_EDGE('',*,*,#16522,.F.);
#23285=ORIENTED_EDGE('',*,*,#16570,.F.);
#23286=ORIENTED_EDGE('',*,*,#16571,.F.);
#23287=ORIENTED_EDGE('',*,*,#16527,.F.);
#23288=ORIENTED_EDGE('',*,*,#16572,.T.);
#23289=ORIENTED_EDGE('',*,*,#16573,.T.);
#23290=ORIENTED_EDGE('',*,*,#16574,.T.);
#23291=ORIENTED_EDGE('',*,*,#16568,.T.);
#23292=ORIENTED_EDGE('',*,*,#16526,.F.);
#23293=ORIENTED_EDGE('',*,*,#16509,.T.);
#23294=ORIENTED_EDGE('',*,*,#16506,.T.);
#23295=ORIENTED_EDGE('',*,*,#16575,.T.);
#23296=ORIENTED_EDGE('',*,*,#16572,.F.);
#23297=ORIENTED_EDGE('',*,*,#16573,.F.);
#23298=ORIENTED_EDGE('',*,*,#16575,.F.);
#23299=ORIENTED_EDGE('',*,*,#16505,.T.);
#23300=ORIENTED_EDGE('',*,*,#16485,.T.);
#23301=ORIENTED_EDGE('',*,*,#16500,.F.);
#23302=ORIENTED_EDGE('',*,*,#16501,.T.);
#23303=ORIENTED_EDGE('',*,*,#16414,.F.);
#23304=ORIENTED_EDGE('',*,*,#16410,.T.);
#23305=ORIENTED_EDGE('',*,*,#16406,.F.);
#23306=ORIENTED_EDGE('',*,*,#16495,.T.);
#23307=ORIENTED_EDGE('',*,*,#16478,.T.);
#23308=ORIENTED_EDGE('',*,*,#16482,.T.);
#23309=ORIENTED_EDGE('',*,*,#16507,.T.);
#23310=ORIENTED_EDGE('',*,*,#16576,.F.);
#23311=ORIENTED_EDGE('',*,*,#16577,.F.);
#23312=ORIENTED_EDGE('',*,*,#16578,.F.);
#23313=ORIENTED_EDGE('',*,*,#16579,.F.);
#23314=ORIENTED_EDGE('',*,*,#16580,.F.);
#23315=ORIENTED_EDGE('',*,*,#16518,.F.);
#23316=ORIENTED_EDGE('',*,*,#16571,.T.);
#23317=ORIENTED_EDGE('',*,*,#16581,.T.);
#23318=ORIENTED_EDGE('',*,*,#16577,.T.);
#23319=ORIENTED_EDGE('',*,*,#16582,.T.);
#23320=ORIENTED_EDGE('',*,*,#16514,.F.);
#23321=ORIENTED_EDGE('',*,*,#16582,.F.);
#23322=ORIENTED_EDGE('',*,*,#16576,.T.);
#23323=ORIENTED_EDGE('',*,*,#16508,.F.);
#23324=ORIENTED_EDGE('',*,*,#16513,.T.);
#23325=ORIENTED_EDGE('',*,*,#16458,.F.);
#23326=ORIENTED_EDGE('',*,*,#16583,.T.);
#23327=ORIENTED_EDGE('',*,*,#16584,.T.);
#23328=ORIENTED_EDGE('',*,*,#16585,.T.);
#23329=ORIENTED_EDGE('',*,*,#16586,.T.);
#23330=ORIENTED_EDGE('',*,*,#16457,.F.);
#23331=ORIENTED_EDGE('',*,*,#16451,.T.);
#23332=ORIENTED_EDGE('',*,*,#16439,.T.);
#23333=ORIENTED_EDGE('',*,*,#16587,.T.);
#23334=ORIENTED_EDGE('',*,*,#16583,.F.);
#23335=ORIENTED_EDGE('',*,*,#16584,.F.);
#23336=ORIENTED_EDGE('',*,*,#16587,.F.);
#23337=ORIENTED_EDGE('',*,*,#16438,.T.);
#23338=ORIENTED_EDGE('',*,*,#16431,.T.);
#23339=ORIENTED_EDGE('',*,*,#16428,.F.);
#23340=ORIENTED_EDGE('',*,*,#16588,.T.);
#23341=ORIENTED_EDGE('',*,*,#16418,.F.);
#23342=ORIENTED_EDGE('',*,*,#16422,.T.);
#23343=ORIENTED_EDGE('',*,*,#16423,.F.);
#23344=ORIENTED_EDGE('',*,*,#16450,.T.);
#23345=ORIENTED_EDGE('',*,*,#16440,.T.);
#23346=ORIENTED_EDGE('',*,*,#16435,.T.);
#23347=ORIENTED_EDGE('',*,*,#16444,.T.);
#23348=ORIENTED_EDGE('',*,*,#16473,.F.);
#23349=ORIENTED_EDGE('',*,*,#16476,.F.);
#23350=ORIENTED_EDGE('',*,*,#16589,.F.);
#23351=ORIENTED_EDGE('',*,*,#16590,.F.);
#23352=ORIENTED_EDGE('',*,*,#16591,.F.);
#23353=ORIENTED_EDGE('',*,*,#16470,.F.);
#23354=ORIENTED_EDGE('',*,*,#16592,.F.);
#23355=ORIENTED_EDGE('',*,*,#16593,.F.);
#23356=ORIENTED_EDGE('',*,*,#16474,.F.);
#23357=ORIENTED_EDGE('',*,*,#16469,.F.);
#23358=ORIENTED_EDGE('',*,*,#16463,.T.);
#23359=ORIENTED_EDGE('',*,*,#16594,.T.);
#23360=ORIENTED_EDGE('',*,*,#16595,.T.);
#23361=ORIENTED_EDGE('',*,*,#16592,.T.);
#23362=ORIENTED_EDGE('',*,*,#16459,.F.);
#23363=ORIENTED_EDGE('',*,*,#16586,.F.);
#23364=ORIENTED_EDGE('',*,*,#16596,.F.);
#23365=ORIENTED_EDGE('',*,*,#16465,.F.);
#23366=ORIENTED_EDGE('',*,*,#16597,.T.);
#23367=ORIENTED_EDGE('',*,*,#16598,.T.);
#23368=ORIENTED_EDGE('',*,*,#16599,.T.);
#23369=ORIENTED_EDGE('',*,*,#16598,.F.);
#23370=ORIENTED_EDGE('',*,*,#16600,.F.);
#23371=ORIENTED_EDGE('',*,*,#16601,.T.);
#23372=ORIENTED_EDGE('',*,*,#16599,.F.);
#23373=ORIENTED_EDGE('',*,*,#16601,.F.);
#23374=ORIENTED_EDGE('',*,*,#16467,.F.);
#23375=ORIENTED_EDGE('',*,*,#16602,.F.);
#23376=ORIENTED_EDGE('',*,*,#16594,.F.);
#23377=ORIENTED_EDGE('',*,*,#16462,.F.);
#23378=ORIENTED_EDGE('',*,*,#16603,.F.);
#23379=ORIENTED_EDGE('',*,*,#16597,.F.);
#23380=ORIENTED_EDGE('',*,*,#16590,.T.);
#23381=ORIENTED_EDGE('',*,*,#16604,.T.);
#23382=ORIENTED_EDGE('',*,*,#16600,.T.);
#23383=ORIENTED_EDGE('',*,*,#16604,.F.);
#23384=ORIENTED_EDGE('',*,*,#16579,.T.);
#23385=ORIENTED_EDGE('',*,*,#16605,.T.);
#23386=ORIENTED_EDGE('',*,*,#16606,.T.);
#23387=ORIENTED_EDGE('',*,*,#16605,.F.);
#23388=ORIENTED_EDGE('',*,*,#16607,.F.);
#23389=ORIENTED_EDGE('',*,*,#16608,.T.);
#23390=ORIENTED_EDGE('',*,*,#16606,.F.);
#23391=ORIENTED_EDGE('',*,*,#16608,.F.);
#23392=ORIENTED_EDGE('',*,*,#16609,.T.);
#23393=ORIENTED_EDGE('',*,*,#16610,.T.);
#23394=ORIENTED_EDGE('',*,*,#16607,.T.);
#23395=ORIENTED_EDGE('',*,*,#16610,.F.);
#23396=ORIENTED_EDGE('',*,*,#16532,.F.);
#23397=ORIENTED_EDGE('',*,*,#16611,.F.);
#23398=ORIENTED_EDGE('',*,*,#16520,.F.);
#23399=ORIENTED_EDGE('',*,*,#16525,.F.);
#23400=ORIENTED_EDGE('',*,*,#16612,.F.);
#23401=ORIENTED_EDGE('',*,*,#16609,.F.);
#23402=ORIENTED_EDGE('',*,*,#16603,.T.);
#23403=ORIENTED_EDGE('',*,*,#16613,.T.);
#23404=ORIENTED_EDGE('',*,*,#16614,.T.);
#23405=ORIENTED_EDGE('',*,*,#16613,.F.);
#23406=ORIENTED_EDGE('',*,*,#16615,.F.);
#23407=ORIENTED_EDGE('',*,*,#16616,.T.);
#23408=ORIENTED_EDGE('',*,*,#16614,.F.);
#23409=ORIENTED_EDGE('',*,*,#16616,.F.);
#23410=ORIENTED_EDGE('',*,*,#16591,.T.);
#23411=ORIENTED_EDGE('',*,*,#16617,.T.);
#23412=ORIENTED_EDGE('',*,*,#16615,.T.);
#23413=ORIENTED_EDGE('',*,*,#16617,.F.);
#23414=ORIENTED_EDGE('',*,*,#16580,.T.);
#23415=ORIENTED_EDGE('',*,*,#16618,.T.);
#23416=ORIENTED_EDGE('',*,*,#16619,.T.);
#23417=ORIENTED_EDGE('',*,*,#16618,.F.);
#23418=ORIENTED_EDGE('',*,*,#16620,.F.);
#23419=ORIENTED_EDGE('',*,*,#16621,.T.);
#23420=ORIENTED_EDGE('',*,*,#16619,.F.);
#23421=ORIENTED_EDGE('',*,*,#16621,.F.);
#23422=ORIENTED_EDGE('',*,*,#16612,.T.);
#23423=ORIENTED_EDGE('',*,*,#16622,.T.);
#23424=ORIENTED_EDGE('',*,*,#16620,.T.);
#23425=ORIENTED_EDGE('',*,*,#16622,.F.);
#23426=ORIENTED_EDGE('',*,*,#16566,.T.);
#23427=ORIENTED_EDGE('',*,*,#16623,.T.);
#23428=ORIENTED_EDGE('',*,*,#16624,.T.);
#23429=ORIENTED_EDGE('',*,*,#16623,.F.);
#23430=ORIENTED_EDGE('',*,*,#16624,.F.);
#23431=ORIENTED_EDGE('',*,*,#16625,.T.);
#23432=ORIENTED_EDGE('',*,*,#16626,.F.);
#23433=ORIENTED_EDGE('',*,*,#16625,.F.);
#23434=ORIENTED_EDGE('',*,*,#16567,.T.);
#23435=ORIENTED_EDGE('',*,*,#16627,.T.);
#23436=ORIENTED_EDGE('',*,*,#16628,.T.);
#23437=ORIENTED_EDGE('',*,*,#16627,.F.);
#23438=ORIENTED_EDGE('',*,*,#16628,.F.);
#23439=ORIENTED_EDGE('',*,*,#16629,.T.);
#23440=ORIENTED_EDGE('',*,*,#16630,.F.);
#23441=ORIENTED_EDGE('',*,*,#16629,.F.);
#23442=ORIENTED_EDGE('',*,*,#16447,.T.);
#23443=ORIENTED_EDGE('',*,*,#16631,.T.);
#23444=ORIENTED_EDGE('',*,*,#16632,.T.);
#23445=ORIENTED_EDGE('',*,*,#16633,.T.);
#23446=ORIENTED_EDGE('',*,*,#16634,.T.);
#23447=ORIENTED_EDGE('',*,*,#16635,.T.);
#23448=ORIENTED_EDGE('',*,*,#16632,.F.);
#23449=ORIENTED_EDGE('',*,*,#16636,.T.);
#23450=ORIENTED_EDGE('',*,*,#16637,.T.);
#23451=ORIENTED_EDGE('',*,*,#16638,.T.);
#23452=ORIENTED_EDGE('',*,*,#16634,.F.);
#23453=ORIENTED_EDGE('',*,*,#16639,.T.);
#23454=ORIENTED_EDGE('',*,*,#16640,.T.);
#23455=ORIENTED_EDGE('',*,*,#16641,.T.);
#23456=ORIENTED_EDGE('',*,*,#16637,.F.);
#23457=ORIENTED_EDGE('',*,*,#16642,.T.);
#23458=ORIENTED_EDGE('',*,*,#16503,.F.);
#23459=ORIENTED_EDGE('',*,*,#16643,.T.);
#23460=ORIENTED_EDGE('',*,*,#16640,.F.);
#23461=ORIENTED_EDGE('',*,*,#16644,.T.);
#23462=ORIENTED_EDGE('',*,*,#16644,.F.);
#23463=ORIENTED_EDGE('',*,*,#16642,.F.);
#23464=ORIENTED_EDGE('',*,*,#16639,.F.);
#23465=ORIENTED_EDGE('',*,*,#16636,.F.);
#23466=ORIENTED_EDGE('',*,*,#16631,.F.);
#23467=ORIENTED_EDGE('',*,*,#16446,.T.);
#23468=ORIENTED_EDGE('',*,*,#16424,.F.);
#23469=ORIENTED_EDGE('',*,*,#16420,.T.);
#23470=ORIENTED_EDGE('',*,*,#16416,.F.);
#23471=ORIENTED_EDGE('',*,*,#16645,.T.);
#23472=ORIENTED_EDGE('',*,*,#16646,.F.);
#23473=ORIENTED_EDGE('',*,*,#16647,.F.);
#23474=ORIENTED_EDGE('',*,*,#16648,.F.);
#23475=ORIENTED_EDGE('',*,*,#16649,.F.);
#23476=ORIENTED_EDGE('',*,*,#16650,.F.);
#23477=ORIENTED_EDGE('',*,*,#16491,.T.);
#23478=ORIENTED_EDGE('',*,*,#16408,.F.);
#23479=ORIENTED_EDGE('',*,*,#16412,.T.);
#23480=ORIENTED_EDGE('',*,*,#16413,.F.);
#23481=ORIENTED_EDGE('',*,*,#16504,.T.);
#23482=ORIENTED_EDGE('',*,*,#16651,.F.);
#23483=ORIENTED_EDGE('',*,*,#16578,.T.);
#23484=ORIENTED_EDGE('',*,*,#16581,.F.);
#23485=ORIENTED_EDGE('',*,*,#16570,.T.);
#23486=ORIENTED_EDGE('',*,*,#16521,.F.);
#23487=ORIENTED_EDGE('',*,*,#16611,.T.);
#23488=ORIENTED_EDGE('',*,*,#16531,.F.);
#23489=ORIENTED_EDGE('',*,*,#16569,.T.);
#23490=ORIENTED_EDGE('',*,*,#16574,.F.);
#23491=ORIENTED_EDGE('',*,*,#16593,.T.);
#23492=ORIENTED_EDGE('',*,*,#16595,.F.);
#23493=ORIENTED_EDGE('',*,*,#16602,.T.);
#23494=ORIENTED_EDGE('',*,*,#16466,.F.);
#23495=ORIENTED_EDGE('',*,*,#16596,.T.);
#23496=ORIENTED_EDGE('',*,*,#16585,.F.);
#23497=ORIENTED_EDGE('',*,*,#16589,.T.);
#23498=ORIENTED_EDGE('',*,*,#16475,.F.);
#23499=ORIENTED_EDGE('',*,*,#16652,.F.);
#23500=ORIENTED_EDGE('',*,*,#16492,.T.);
#23501=ORIENTED_EDGE('',*,*,#16650,.T.);
#23502=ORIENTED_EDGE('',*,*,#16653,.T.);
#23503=ORIENTED_EDGE('',*,*,#16654,.T.);
#23504=ORIENTED_EDGE('',*,*,#16655,.T.);
#23505=ORIENTED_EDGE('',*,*,#16656,.T.);
#23506=ORIENTED_EDGE('',*,*,#16653,.F.);
#23507=ORIENTED_EDGE('',*,*,#16649,.T.);
#23508=ORIENTED_EDGE('',*,*,#16657,.T.);
#23509=ORIENTED_EDGE('',*,*,#16658,.T.);
#23510=ORIENTED_EDGE('',*,*,#16655,.F.);
#23511=ORIENTED_EDGE('',*,*,#16648,.T.);
#23512=ORIENTED_EDGE('',*,*,#16659,.T.);
#23513=ORIENTED_EDGE('',*,*,#16660,.T.);
#23514=ORIENTED_EDGE('',*,*,#16657,.F.);
#23515=ORIENTED_EDGE('',*,*,#16647,.T.);
#23516=ORIENTED_EDGE('',*,*,#16661,.F.);
#23517=ORIENTED_EDGE('',*,*,#16662,.T.);
#23518=ORIENTED_EDGE('',*,*,#16659,.F.);
#23519=ORIENTED_EDGE('',*,*,#16646,.T.);
#23520=ORIENTED_EDGE('',*,*,#16652,.T.);
#23521=ORIENTED_EDGE('',*,*,#16663,.T.);
#23522=ORIENTED_EDGE('',*,*,#16630,.T.);
#23523=ORIENTED_EDGE('',*,*,#16663,.F.);
#23524=ORIENTED_EDGE('',*,*,#16651,.T.);
#23525=ORIENTED_EDGE('',*,*,#16664,.T.);
#23526=ORIENTED_EDGE('',*,*,#16626,.T.);
#23527=ORIENTED_EDGE('',*,*,#16664,.F.);
#23528=ORIENTED_EDGE('',*,*,#16430,.F.);
#23529=ORIENTED_EDGE('',*,*,#16437,.F.);
#23530=ORIENTED_EDGE('',*,*,#16443,.F.);
#23531=ORIENTED_EDGE('',*,*,#16665,.F.);
#23532=ORIENTED_EDGE('',*,*,#16426,.F.);
#23533=ORIENTED_EDGE('',*,*,#16665,.T.);
#23534=ORIENTED_EDGE('',*,*,#16442,.F.);
#23535=ORIENTED_EDGE('',*,*,#16449,.F.);
#23536=ORIENTED_EDGE('',*,*,#16666,.F.);
#23537=ORIENTED_EDGE('',*,*,#16667,.F.);
#23538=ORIENTED_EDGE('',*,*,#16419,.F.);
#23539=ORIENTED_EDGE('',*,*,#16588,.F.);
#23540=ORIENTED_EDGE('',*,*,#16427,.F.);
#23541=ORIENTED_EDGE('',*,*,#16667,.T.);
#23542=ORIENTED_EDGE('',*,*,#16668,.T.);
#23543=ORIENTED_EDGE('',*,*,#16661,.T.);
#23544=ORIENTED_EDGE('',*,*,#16645,.F.);
#23545=ORIENTED_EDGE('',*,*,#16635,.F.);
#23546=ORIENTED_EDGE('',*,*,#16669,.T.);
#23547=ORIENTED_EDGE('',*,*,#16565,.T.);
#23548=ORIENTED_EDGE('',*,*,#16670,.T.);
#23549=ORIENTED_EDGE('',*,*,#16638,.F.);
#23550=ORIENTED_EDGE('',*,*,#16671,.T.);
#23551=ORIENTED_EDGE('',*,*,#16563,.T.);
#23552=ORIENTED_EDGE('',*,*,#16669,.F.);
#23553=ORIENTED_EDGE('',*,*,#16641,.F.);
#23554=ORIENTED_EDGE('',*,*,#16672,.T.);
#23555=ORIENTED_EDGE('',*,*,#16561,.T.);
#23556=ORIENTED_EDGE('',*,*,#16671,.F.);
#23557=ORIENTED_EDGE('',*,*,#16502,.F.);
#23558=ORIENTED_EDGE('',*,*,#16496,.T.);
#23559=ORIENTED_EDGE('',*,*,#16493,.F.);
#23560=ORIENTED_EDGE('',*,*,#16654,.F.);
#23561=ORIENTED_EDGE('',*,*,#16673,.T.);
#23562=ORIENTED_EDGE('',*,*,#16558,.T.);
#23563=ORIENTED_EDGE('',*,*,#16672,.F.);
#23564=ORIENTED_EDGE('',*,*,#16643,.F.);
#23565=ORIENTED_EDGE('',*,*,#16656,.F.);
#23566=ORIENTED_EDGE('',*,*,#16674,.T.);
#23567=ORIENTED_EDGE('',*,*,#16675,.T.);
#23568=ORIENTED_EDGE('',*,*,#16673,.F.);
#23569=ORIENTED_EDGE('',*,*,#16658,.F.);
#23570=ORIENTED_EDGE('',*,*,#16676,.T.);
#23571=ORIENTED_EDGE('',*,*,#16677,.T.);
#23572=ORIENTED_EDGE('',*,*,#16674,.F.);
#23573=ORIENTED_EDGE('',*,*,#16660,.F.);
#23574=ORIENTED_EDGE('',*,*,#16678,.T.);
#23575=ORIENTED_EDGE('',*,*,#16679,.T.);
#23576=ORIENTED_EDGE('',*,*,#16676,.F.);
#23577=ORIENTED_EDGE('',*,*,#16633,.F.);
#23578=ORIENTED_EDGE('',*,*,#16670,.F.);
#23579=ORIENTED_EDGE('',*,*,#16680,.T.);
#23580=ORIENTED_EDGE('',*,*,#16678,.F.);
#23581=ORIENTED_EDGE('',*,*,#16662,.F.);
#23582=ORIENTED_EDGE('',*,*,#16668,.F.);
#23583=ORIENTED_EDGE('',*,*,#16666,.T.);
#23584=ORIENTED_EDGE('',*,*,#16448,.F.);
#23585=ORIENTED_EDGE('',*,*,#16544,.F.);
#23586=ORIENTED_EDGE('',*,*,#16681,.F.);
#23587=ORIENTED_EDGE('',*,*,#16677,.F.);
#23588=ORIENTED_EDGE('',*,*,#16682,.F.);
#23589=ORIENTED_EDGE('',*,*,#16541,.F.);
#23590=ORIENTED_EDGE('',*,*,#16682,.T.);
#23591=ORIENTED_EDGE('',*,*,#16679,.F.);
#23592=ORIENTED_EDGE('',*,*,#16683,.T.);
#23593=ORIENTED_EDGE('',*,*,#16538,.F.);
#23594=ORIENTED_EDGE('',*,*,#16683,.F.);
#23595=ORIENTED_EDGE('',*,*,#16680,.F.);
#23596=ORIENTED_EDGE('',*,*,#16564,.F.);
#23597=ORIENTED_EDGE('',*,*,#16547,.F.);
#23598=ORIENTED_EDGE('',*,*,#16559,.T.);
#23599=ORIENTED_EDGE('',*,*,#16675,.F.);
#23600=ORIENTED_EDGE('',*,*,#16681,.T.);
#26675=PLANE('',#30014);
#26676=PLANE('',#30015);
#26677=PLANE('',#30016);
#26678=PLANE('',#30017);
#26679=PLANE('',#30018);
#26680=PLANE('',#30019);
#26681=PLANE('',#30020);
#26682=PLANE('',#30021);
#26683=PLANE('',#30022);
#26684=PLANE('',#30023);
#26685=PLANE('',#30024);
#26686=PLANE('',#30025);
#26687=PLANE('',#30026);
#26688=PLANE('',#30027);
#26689=PLANE('',#30028);
#26690=PLANE('',#30029);
#26691=PLANE('',#30030);
#26692=PLANE('',#30031);
#26693=PLANE('',#30032);
#26694=PLANE('',#30033);
#26695=PLANE('',#30034);
#26696=PLANE('',#30035);
#26697=PLANE('',#30036);
#26698=PLANE('',#30037);
#26699=PLANE('',#30038);
#26700=PLANE('',#30039);
#26701=PLANE('',#30040);
#26702=PLANE('',#30041);
#26703=PLANE('',#30042);
#26704=PLANE('',#30043);
#26705=PLANE('',#30044);
#26706=PLANE('',#30045);
#26707=PLANE('',#30046);
#26708=PLANE('',#30047);
#26709=PLANE('',#30051);
#26710=PLANE('',#30055);
#26711=PLANE('',#30059);
#26712=PLANE('',#30063);
#26713=PLANE('',#30064);
#26714=PLANE('',#30067);
#26715=PLANE('',#30070);
#26716=PLANE('',#30073);
#26717=PLANE('',#30074);
#26718=PLANE('',#30075);
#26719=PLANE('',#30076);
#26720=PLANE('',#30077);
#26721=PLANE('',#30080);
#26722=PLANE('',#30081);
#26723=PLANE('',#30082);
#26724=PLANE('',#30083);
#26725=PLANE('',#30084);
#26726=PLANE('',#30087);
#26727=PLANE('',#30088);
#26728=PLANE('',#30089);
#26729=PLANE('',#30095);
#26730=PLANE('',#30104);
#26731=PLANE('',#30124);
#26732=PLANE('',#30128);
#26733=PLANE('',#30132);
#26734=PLANE('',#30133);
#26735=PLANE('',#30138);
#26736=PLANE('',#30141);
#26737=PLANE('',#30144);
#26738=PLANE('',#30147);
#26739=PLANE('',#30148);
#26740=PLANE('',#30149);
#26741=PLANE('',#30151);
#26742=PLANE('',#30153);
#26743=PLANE('',#30156);
#26744=PLANE('',#30159);
#26745=PLANE('',#30160);
#26746=PLANE('',#30162);
#27872=ADVANCED_FACE('',(#3964),#26675,.T.);
#27873=ADVANCED_FACE('',(#3965),#26676,.T.);
#27874=ADVANCED_FACE('',(#3966),#26677,.T.);
#27875=ADVANCED_FACE('',(#3967),#26678,.T.);
#27876=ADVANCED_FACE('',(#3968),#26679,.T.);
#27877=ADVANCED_FACE('',(#3969),#26680,.T.);
#27878=ADVANCED_FACE('',(#3970),#26681,.T.);
#27879=ADVANCED_FACE('',(#3971),#26682,.T.);
#27880=ADVANCED_FACE('',(#3972),#26683,.T.);
#27881=ADVANCED_FACE('',(#3973),#26684,.T.);
#27882=ADVANCED_FACE('',(#3974),#26685,.T.);
#27883=ADVANCED_FACE('',(#3975),#26686,.T.);
#27884=ADVANCED_FACE('',(#3976),#26687,.T.);
#27885=ADVANCED_FACE('',(#3977),#26688,.T.);
#27886=ADVANCED_FACE('',(#3978),#26689,.T.);
#27887=ADVANCED_FACE('',(#3979),#26690,.T.);
#27888=ADVANCED_FACE('',(#3980),#26691,.T.);
#27889=ADVANCED_FACE('',(#3981),#26692,.T.);
#27890=ADVANCED_FACE('',(#3982),#26693,.T.);
#27891=ADVANCED_FACE('',(#3983),#26694,.T.);
#27892=ADVANCED_FACE('',(#3984),#26695,.T.);
#27893=ADVANCED_FACE('',(#3985),#26696,.T.);
#27894=ADVANCED_FACE('',(#3986),#26697,.T.);
#27895=ADVANCED_FACE('',(#3987),#26698,.T.);
#27896=ADVANCED_FACE('',(#3988),#26699,.T.);
#27897=ADVANCED_FACE('',(#3989),#26700,.T.);
#27898=ADVANCED_FACE('',(#3990),#26701,.T.);
#27899=ADVANCED_FACE('',(#3991),#26702,.T.);
#27900=ADVANCED_FACE('',(#3992),#26703,.T.);
#27901=ADVANCED_FACE('',(#3993),#26704,.T.);
#27902=ADVANCED_FACE('',(#3994),#26705,.T.);
#27903=ADVANCED_FACE('',(#3995),#26706,.T.);
#27904=ADVANCED_FACE('',(#3996),#26707,.T.);
#27905=ADVANCED_FACE('',(#3997),#26708,.T.);
#27906=ADVANCED_FACE('',(#3998),#2865,.T.);
#27907=ADVANCED_FACE('',(#3999),#26709,.T.);
#27908=ADVANCED_FACE('',(#4000),#2866,.T.);
#27909=ADVANCED_FACE('',(#4001),#26710,.T.);
#27910=ADVANCED_FACE('',(#4002),#2867,.T.);
#27911=ADVANCED_FACE('',(#4003),#26711,.T.);
#27912=ADVANCED_FACE('',(#4004),#2868,.T.);
#27913=ADVANCED_FACE('',(#4005),#26712,.T.);
#27914=ADVANCED_FACE('',(#4006),#26713,.T.);
#27915=ADVANCED_FACE('',(#4007),#1672,.T.);
#27916=ADVANCED_FACE('',(#4008),#26714,.T.);
#27917=ADVANCED_FACE('',(#4009),#1673,.T.);
#27918=ADVANCED_FACE('',(#4010,#1953,#1954),#26715,.F.);
#27919=ADVANCED_FACE('',(#4011),#26716,.T.);
#27920=ADVANCED_FACE('',(#4012),#26717,.T.);
#27921=ADVANCED_FACE('',(#4013),#26718,.T.);
#27922=ADVANCED_FACE('',(#4014),#26719,.T.);
#27923=ADVANCED_FACE('',(#4015,#1955,#1956),#26720,.T.);
#27924=ADVANCED_FACE('',(#4016),#26721,.T.);
#27925=ADVANCED_FACE('',(#4017),#26722,.T.);
#27926=ADVANCED_FACE('',(#4018),#26723,.T.);
#27927=ADVANCED_FACE('',(#4019),#26724,.T.);
#27928=ADVANCED_FACE('',(#4020,#1957,#1958),#26725,.T.);
#27929=ADVANCED_FACE('',(#4021),#26726,.T.);
#27930=ADVANCED_FACE('',(#4022),#26727,.T.);
#27931=ADVANCED_FACE('',(#4023),#26728,.T.);
#27932=ADVANCED_FACE('',(#4024),#2869,.F.);
#27933=ADVANCED_FACE('',(#4025),#1674,.F.);
#27934=ADVANCED_FACE('',(#4026,#1959,#1960),#26729,.T.);
#27935=ADVANCED_FACE('',(#4027),#2870,.F.);
#27936=ADVANCED_FACE('',(#4028),#2871,.F.);
#27937=ADVANCED_FACE('',(#4029),#1675,.F.);
#27938=ADVANCED_FACE('',(#4030),#2872,.F.);
#27939=ADVANCED_FACE('',(#4031,#1961,#1962),#26730,.T.);
#27940=ADVANCED_FACE('',(#4032),#2873,.F.);
#27941=ADVANCED_FACE('',(#4033),#1676,.F.);
#27942=ADVANCED_FACE('',(#4034),#2874,.F.);
#27943=ADVANCED_FACE('',(#4035),#2875,.F.);
#27944=ADVANCED_FACE('',(#4036),#1677,.F.);
#27945=ADVANCED_FACE('',(#4037),#2876,.F.);
#27946=ADVANCED_FACE('',(#4038),#2877,.F.);
#27947=ADVANCED_FACE('',(#4039),#1678,.F.);
#27948=ADVANCED_FACE('',(#4040),#2878,.F.);
#27949=ADVANCED_FACE('',(#4041),#1679,.F.);
#27950=ADVANCED_FACE('',(#4042),#26731,.T.);
#27951=ADVANCED_FACE('',(#4043),#2879,.T.);
#27952=ADVANCED_FACE('',(#4044),#26732,.T.);
#27953=ADVANCED_FACE('',(#4045),#2880,.T.);
#27954=ADVANCED_FACE('',(#4046),#26733,.T.);
#27955=ADVANCED_FACE('',(#4047,#1963,#1964,#1965,#1966),#26734,.T.);
#27956=ADVANCED_FACE('',(#4048),#26735,.T.);
#27957=ADVANCED_FACE('',(#4049),#2881,.T.);
#27958=ADVANCED_FACE('',(#4050),#26736,.T.);
#27959=ADVANCED_FACE('',(#4051),#2882,.T.);
#27960=ADVANCED_FACE('',(#4052),#26737,.T.);
#27961=ADVANCED_FACE('',(#4053),#2883,.F.);
#27962=ADVANCED_FACE('',(#4054),#2884,.F.);
#27963=ADVANCED_FACE('',(#4055),#26738,.T.);
#27964=ADVANCED_FACE('',(#4056),#26739,.T.);
#27965=ADVANCED_FACE('',(#4057),#26740,.T.);
#27966=ADVANCED_FACE('',(#4058),#2885,.T.);
#27967=ADVANCED_FACE('',(#4059),#26741,.T.);
#27968=ADVANCED_FACE('',(#4060),#2886,.T.);
#27969=ADVANCED_FACE('',(#4061),#26742,.T.);
#27970=ADVANCED_FACE('',(#4062),#2887,.T.);
#27971=ADVANCED_FACE('',(#4063),#26743,.T.);
#27972=ADVANCED_FACE('',(#4064),#2888,.T.);
#27973=ADVANCED_FACE('',(#4065),#26744,.T.);
#27974=ADVANCED_FACE('',(#4066),#26745,.T.);
#27975=ADVANCED_FACE('',(#4067),#1680,.T.);
#27976=ADVANCED_FACE('',(#4068),#26746,.T.);
#27977=ADVANCED_FACE('',(#4069),#1681,.T.);
#28469=CLOSED_SHELL('',(#27872,#27873,#27874,#27875,#27876,#27877,#27878,
#27879,#27880,#27881,#27882,#27883,#27884,#27885,#27886,#27887,#27888,#27889,
#27890,#27891,#27892,#27893,#27894,#27895,#27896,#27897,#27898,#27899,#27900,
#27901,#27902,#27903,#27904,#27905,#27906,#27907,#27908,#27909,#27910,#27911,
#27912,#27913,#27914,#27915,#27916,#27917,#27918,#27919,#27920,#27921,#27922,
#27923,#27924,#27925,#27926,#27927,#27928,#27929,#27930,#27931,#27932,#27933,
#27934,#27935,#27936,#27937,#27938,#27939,#27940,#27941,#27942,#27943,#27944,
#27945,#27946,#27947,#27948,#27949,#27950,#27951,#27952,#27953,#27954,#27955,
#27956,#27957,#27958,#27959,#27960,#27961,#27962,#27963,#27964,#27965,#27966,
#27967,#27968,#27969,#27970,#27971,#27972,#27973,#27974,#27975,#27976,#27977));
#30013=AXIS2_PLACEMENT_3D('',#50002,#35211,#35212);
#30014=AXIS2_PLACEMENT_3D('',#50003,#35213,#35214);
#30015=AXIS2_PLACEMENT_3D('',#50012,#35219,#35220);
#30016=AXIS2_PLACEMENT_3D('',#50018,#35224,#35225);
#30017=AXIS2_PLACEMENT_3D('',#50024,#35229,#35230);
#30018=AXIS2_PLACEMENT_3D('',#50033,#35235,#35236);
#30019=AXIS2_PLACEMENT_3D('',#50039,#35240,#35241);
#30020=AXIS2_PLACEMENT_3D('',#50045,#35245,#35246);
#30021=AXIS2_PLACEMENT_3D('',#50056,#35252,#35253);
#30022=AXIS2_PLACEMENT_3D('',#50070,#35261,#35262);
#30023=AXIS2_PLACEMENT_3D('',#50074,#35265,#35266);
#30024=AXIS2_PLACEMENT_3D('',#50082,#35271,#35272);
#30025=AXIS2_PLACEMENT_3D('',#50086,#35275,#35276);
#30026=AXIS2_PLACEMENT_3D('',#50095,#35282,#35283);
#30027=AXIS2_PLACEMENT_3D('',#50105,#35289,#35290);
#30028=AXIS2_PLACEMENT_3D('',#50115,#35296,#35297);
#30029=AXIS2_PLACEMENT_3D('',#50123,#35302,#35303);
#30030=AXIS2_PLACEMENT_3D('',#50129,#35307,#35308);
#30031=AXIS2_PLACEMENT_3D('',#50137,#35313,#35314);
#30032=AXIS2_PLACEMENT_3D('',#50141,#35317,#35318);
#30033=AXIS2_PLACEMENT_3D('',#50147,#35322,#35323);
#30034=AXIS2_PLACEMENT_3D('',#50158,#35329,#35330);
#30035=AXIS2_PLACEMENT_3D('',#50172,#35338,#35339);
#30036=AXIS2_PLACEMENT_3D('',#50176,#35342,#35343);
#30037=AXIS2_PLACEMENT_3D('',#50185,#35349,#35350);
#30038=AXIS2_PLACEMENT_3D('',#50191,#35354,#35355);
#30039=AXIS2_PLACEMENT_3D('',#50195,#35358,#35359);
#30040=AXIS2_PLACEMENT_3D('',#50202,#35364,#35365);
#30041=AXIS2_PLACEMENT_3D('',#50206,#35368,#35369);
#30042=AXIS2_PLACEMENT_3D('',#50210,#35372,#35373);
#30043=AXIS2_PLACEMENT_3D('',#50220,#35379,#35380);
#30044=AXIS2_PLACEMENT_3D('',#50230,#35386,#35387);
#30045=AXIS2_PLACEMENT_3D('',#50238,#35392,#35393);
#30046=AXIS2_PLACEMENT_3D('',#50244,#35397,#35398);
#30047=AXIS2_PLACEMENT_3D('',#50252,#35403,#35404);
#30048=AXIS2_PLACEMENT_3D('',#50258,#35408,#35409);
#30049=AXIS2_PLACEMENT_3D('',#50263,#35411,#35412);
#30050=AXIS2_PLACEMENT_3D('',#50266,#35414,#35415);
#30051=AXIS2_PLACEMENT_3D('',#50267,#35416,#35417);
#30052=AXIS2_PLACEMENT_3D('',#50273,#35421,#35422);
#30053=AXIS2_PLACEMENT_3D('',#50277,#35424,#35425);
#30054=AXIS2_PLACEMENT_3D('',#50278,#35426,#35427);
#30055=AXIS2_PLACEMENT_3D('',#50279,#35428,#35429);
#30056=AXIS2_PLACEMENT_3D('',#50285,#35433,#35434);
#30057=AXIS2_PLACEMENT_3D('',#50289,#35436,#35437);
#30058=AXIS2_PLACEMENT_3D('',#50290,#35438,#35439);
#30059=AXIS2_PLACEMENT_3D('',#50291,#35440,#35441);
#30060=AXIS2_PLACEMENT_3D('',#50297,#35445,#35446);
#30061=AXIS2_PLACEMENT_3D('',#50301,#35448,#35449);
#30062=AXIS2_PLACEMENT_3D('',#50302,#35450,#35451);
#30063=AXIS2_PLACEMENT_3D('',#50303,#35452,#35453);
#30064=AXIS2_PLACEMENT_3D('',#50306,#35456,#35457);
#30065=AXIS2_PLACEMENT_3D('',#50312,#35461,#35462);
#30066=AXIS2_PLACEMENT_3D('',#50315,#35464,#35465);
#30067=AXIS2_PLACEMENT_3D('',#50316,#35466,#35467);
#30068=AXIS2_PLACEMENT_3D('',#50320,#35470,#35471);
#30069=AXIS2_PLACEMENT_3D('',#50323,#35473,#35474);
#30070=AXIS2_PLACEMENT_3D('',#50324,#35475,#35476);
#30071=AXIS2_PLACEMENT_3D('',#50326,#35477,#35478);
#30072=AXIS2_PLACEMENT_3D('',#50328,#35479,#35480);
#30073=AXIS2_PLACEMENT_3D('',#50329,#35481,#35482);
#30074=AXIS2_PLACEMENT_3D('',#50333,#35485,#35486);
#30075=AXIS2_PLACEMENT_3D('',#50337,#35489,#35490);
#30076=AXIS2_PLACEMENT_3D('',#50343,#35494,#35495);
#30077=AXIS2_PLACEMENT_3D('',#50345,#35497,#35498);
#30078=AXIS2_PLACEMENT_3D('',#50352,#35502,#35503);
#30079=AXIS2_PLACEMENT_3D('',#50354,#35504,#35505);
#30080=AXIS2_PLACEMENT_3D('',#50355,#35506,#35507);
#30081=AXIS2_PLACEMENT_3D('',#50358,#35510,#35511);
#30082=AXIS2_PLACEMENT_3D('',#50359,#35512,#35513);
#30083=AXIS2_PLACEMENT_3D('',#50367,#35518,#35519);
#30084=AXIS2_PLACEMENT_3D('',#50369,#35521,#35522);
#30085=AXIS2_PLACEMENT_3D('',#50373,#35525,#35526);
#30086=AXIS2_PLACEMENT_3D('',#50375,#35527,#35528);
#30087=AXIS2_PLACEMENT_3D('',#50376,#35529,#35530);
#30088=AXIS2_PLACEMENT_3D('',#50380,#35533,#35534);
#30089=AXIS2_PLACEMENT_3D('',#50384,#35537,#35538);
#30090=AXIS2_PLACEMENT_3D('',#50386,#35540,#35541);
#30091=AXIS2_PLACEMENT_3D('',#50388,#35542,#35543);
#30092=AXIS2_PLACEMENT_3D('',#50391,#35545,#35546);
#30093=AXIS2_PLACEMENT_3D('',#50392,#35547,#35548);
#30094=AXIS2_PLACEMENT_3D('',#50394,#35549,#35550);
#30095=AXIS2_PLACEMENT_3D('',#50396,#35552,#35553);
#30096=AXIS2_PLACEMENT_3D('',#50399,#35555,#35556);
#30097=AXIS2_PLACEMENT_3D('',#50400,#35557,#35558);
#30098=AXIS2_PLACEMENT_3D('',#50402,#35560,#35561);
#30099=AXIS2_PLACEMENT_3D('',#50405,#35563,#35564);
#30100=AXIS2_PLACEMENT_3D('',#50406,#35565,#35566);
#30101=AXIS2_PLACEMENT_3D('',#50408,#35567,#35568);
#30102=AXIS2_PLACEMENT_3D('',#50410,#35570,#35571);
#30103=AXIS2_PLACEMENT_3D('',#50412,#35572,#35573);
#30104=AXIS2_PLACEMENT_3D('',#50414,#35575,#35576);
#30105=AXIS2_PLACEMENT_3D('',#50417,#35578,#35579);
#30106=AXIS2_PLACEMENT_3D('',#50418,#35580,#35581);
#30107=AXIS2_PLACEMENT_3D('',#50421,#35583,#35584);
#30108=AXIS2_PLACEMENT_3D('',#50422,#35585,#35586);
#30109=AXIS2_PLACEMENT_3D('',#50424,#35587,#35588);
#30110=AXIS2_PLACEMENT_3D('',#50426,#35590,#35591);
#30111=AXIS2_PLACEMENT_3D('',#50428,#35593,#35594);
#30112=AXIS2_PLACEMENT_3D('',#50431,#35596,#35597);
#30113=AXIS2_PLACEMENT_3D('',#50432,#35598,#35599);
#30114=AXIS2_PLACEMENT_3D('',#50434,#35600,#35601);
#30115=AXIS2_PLACEMENT_3D('',#50436,#35603,#35604);
#30116=AXIS2_PLACEMENT_3D('',#50438,#35606,#35607);
#30117=AXIS2_PLACEMENT_3D('',#50441,#35609,#35610);
#30118=AXIS2_PLACEMENT_3D('',#50442,#35611,#35612);
#30119=AXIS2_PLACEMENT_3D('',#50445,#35614,#35615);
#30120=AXIS2_PLACEMENT_3D('',#50446,#35616,#35617);
#30121=AXIS2_PLACEMENT_3D('',#50449,#35619,#35620);
#30122=AXIS2_PLACEMENT_3D('',#50450,#35621,#35622);
#30123=AXIS2_PLACEMENT_3D('',#50453,#35624,#35625);
#30124=AXIS2_PLACEMENT_3D('',#50454,#35626,#35627);
#30125=AXIS2_PLACEMENT_3D('',#50460,#35631,#35632);
#30126=AXIS2_PLACEMENT_3D('',#50464,#35634,#35635);
#30127=AXIS2_PLACEMENT_3D('',#50465,#35636,#35637);
#30128=AXIS2_PLACEMENT_3D('',#50466,#35638,#35639);
#30129=AXIS2_PLACEMENT_3D('',#50472,#35643,#35644);
#30130=AXIS2_PLACEMENT_3D('',#50476,#35646,#35647);
#30131=AXIS2_PLACEMENT_3D('',#50477,#35648,#35649);
#30132=AXIS2_PLACEMENT_3D('',#50478,#35650,#35651);
#30133=AXIS2_PLACEMENT_3D('',#50481,#35654,#35655);
#30134=AXIS2_PLACEMENT_3D('',#50487,#35658,#35659);
#30135=AXIS2_PLACEMENT_3D('',#50491,#35661,#35662);
#30136=AXIS2_PLACEMENT_3D('',#50494,#35664,#35665);
#30137=AXIS2_PLACEMENT_3D('',#50496,#35666,#35667);
#30138=AXIS2_PLACEMENT_3D('',#50497,#35668,#35669);
#30139=AXIS2_PLACEMENT_3D('',#50501,#35672,#35673);
#30140=AXIS2_PLACEMENT_3D('',#50504,#35675,#35676);
#30141=AXIS2_PLACEMENT_3D('',#50505,#35677,#35678);
#30142=AXIS2_PLACEMENT_3D('',#50509,#35681,#35682);
#30143=AXIS2_PLACEMENT_3D('',#50512,#35684,#35685);
#30144=AXIS2_PLACEMENT_3D('',#50513,#35686,#35687);
#30145=AXIS2_PLACEMENT_3D('',#50517,#35690,#35691);
#30146=AXIS2_PLACEMENT_3D('',#50519,#35693,#35694);
#30147=AXIS2_PLACEMENT_3D('',#50521,#35696,#35697);
#30148=AXIS2_PLACEMENT_3D('',#50523,#35699,#35700);
#30149=AXIS2_PLACEMENT_3D('',#50527,#35703,#35704);
#30150=AXIS2_PLACEMENT_3D('',#50529,#35706,#35707);
#30151=AXIS2_PLACEMENT_3D('',#50532,#35710,#35711);
#30152=AXIS2_PLACEMENT_3D('',#50534,#35713,#35714);
#30153=AXIS2_PLACEMENT_3D('',#50536,#35716,#35717);
#30154=AXIS2_PLACEMENT_3D('',#50538,#35719,#35720);
#30155=AXIS2_PLACEMENT_3D('',#50541,#35722,#35723);
#30156=AXIS2_PLACEMENT_3D('',#50542,#35724,#35725);
#30157=AXIS2_PLACEMENT_3D('',#50546,#35728,#35729);
#30158=AXIS2_PLACEMENT_3D('',#50549,#35731,#35732);
#30159=AXIS2_PLACEMENT_3D('',#50550,#35733,#35734);
#30160=AXIS2_PLACEMENT_3D('',#50552,#35736,#35737);
#30161=AXIS2_PLACEMENT_3D('',#50555,#35740,#35741);
#30162=AXIS2_PLACEMENT_3D('',#50557,#35743,#35744);
#30163=AXIS2_PLACEMENT_3D('',#50558,#35745,#35746);
#35211=DIRECTION('axis',(0.,0.,1.));
#35212=DIRECTION('refdir',(1.,0.,0.));
#35213=DIRECTION('center_axis',(0.707106781186547,-0.542827373086154,-0.453142850576268));
#35214=DIRECTION('ref_axis',(-0.53955578700857,0.,-0.841949851657189));
#35215=DIRECTION('',(0.53955578700857,0.,0.841949851657189));
#35216=DIRECTION('',(0.,0.640840764977362,-0.767673833045799));
#35217=DIRECTION('',(-0.608934580549686,-0.793220446414978,0.));
#35218=DIRECTION('',(0.,-0.640840764977362,0.767673833045799));
#35219=DIRECTION('center_axis',(0.,-0.767673833045799,-0.640840764977362));
#35220=DIRECTION('ref_axis',(0.,0.640840764977362,-0.767673833045799));
#35221=DIRECTION('',(1.,0.,0.));
#35222=DIRECTION('',(0.,-0.640840764977362,0.767673833045799));
#35223=DIRECTION('',(-1.,0.,0.));
#35224=DIRECTION('center_axis',(-0.707106781186547,-0.542827373086154,-0.453142850576268));
#35225=DIRECTION('ref_axis',(-0.53955578700857,0.,0.841949851657189));
#35226=DIRECTION('',(-0.608934580549686,0.793220446414978,0.));
#35227=DIRECTION('',(0.53955578700857,0.,-0.841949851657189));
#35228=DIRECTION('',(0.,0.640840764977362,-0.767673833045799));
#35229=DIRECTION('center_axis',(0.707106781186545,0.542827373086156,-0.453142850576269));
#35230=DIRECTION('ref_axis',(-0.539555787008572,0.,-0.841949851657188));
#35231=DIRECTION('',(0.608934580549689,-0.793220446414977,0.));
#35232=DIRECTION('',(0.,0.640840764977362,0.767673833045799));
#35233=DIRECTION('',(-0.539555787008572,0.,-0.841949851657188));
#35234=DIRECTION('',(0.,-0.640840764977362,-0.767673833045799));
#35235=DIRECTION('center_axis',(0.,0.767673833045799,-0.640840764977362));
#35236=DIRECTION('ref_axis',(0.,0.640840764977362,0.767673833045799));
#35237=DIRECTION('',(1.,0.,0.));
#35238=DIRECTION('',(0.,-0.640840764977362,-0.767673833045799));
#35239=DIRECTION('',(-1.,0.,0.));
#35240=DIRECTION('center_axis',(-0.707106781186545,0.542827373086156,-0.453142850576269));
#35241=DIRECTION('ref_axis',(-0.539555787008572,0.,0.841949851657188));
#35242=DIRECTION('',(-0.539555787008572,0.,0.841949851657188));
#35243=DIRECTION('',(0.608934580549689,0.793220446414977,0.));
#35244=DIRECTION('',(0.,0.640840764977362,0.767673833045799));
#35245=DIRECTION('center_axis',(0.707106781186551,-0.5337451437584,0.463806124921093));
#35246=DIRECTION('ref_axis',(0.548464086412375,0.,-0.836174112201423));
#35247=DIRECTION('',(0.602464182205077,0.798145919716418,0.));
#35248=DIRECTION('',(0.,0.655920912175122,0.75482962115391));
#35249=DIRECTION('',(0.548464086412375,0.,-0.836174112201423));
#35250=DIRECTION('',(-0.383127220471085,-0.840492156934374,-0.383127220471092));
#35251=DIRECTION('',(0.,-0.655920912175122,-0.75482962115391));
#35252=DIRECTION('center_axis',(0.,-0.414776498746543,0.909923324290327));
#35253=DIRECTION('ref_axis',(1.,0.,0.));
#35254=DIRECTION('',(-1.,0.,0.));
#35255=DIRECTION('',(0.,0.909923324290327,0.414776498746543));
#35256=DIRECTION('',(-1.,0.,0.));
#35257=DIRECTION('',(0.,-0.909923324290327,-0.414776498746543));
#35258=DIRECTION('',(-1.,0.,0.));
#35259=DIRECTION('',(-0.383127220471085,0.840492156934374,0.383127220471092));
#35260=DIRECTION('',(1.,0.,0.));
#35261=DIRECTION('center_axis',(1.,0.,0.));
#35262=DIRECTION('ref_axis',(0.,0.,-1.));
#35263=DIRECTION('',(0.,0.,1.));
#35264=DIRECTION('',(0.,0.707106781186541,0.707106781186554));
#35265=DIRECTION('center_axis',(-0.707106781186551,-0.5337451437584,0.463806124921093));
#35266=DIRECTION('ref_axis',(0.548464086412375,0.,0.836174112201423));
#35267=DIRECTION('',(0.548464086412375,0.,0.836174112201423));
#35268=DIRECTION('',(0.,-0.655920912175122,-0.75482962115391));
#35269=DIRECTION('',(0.602464182205077,-0.798145919716418,0.));
#35270=DIRECTION('',(0.,0.655920912175122,0.75482962115391));
#35271=DIRECTION('center_axis',(-1.,0.,0.));
#35272=DIRECTION('ref_axis',(0.,0.,1.));
#35273=DIRECTION('',(0.,0.,-1.));
#35274=DIRECTION('',(0.,-0.707106781186541,-0.707106781186554));
#35275=DIRECTION('center_axis',(-1.,0.,0.));
#35276=DIRECTION('ref_axis',(0.,0.,1.));
#35277=DIRECTION('',(0.,1.,0.));
#35278=DIRECTION('',(0.,-0.923879532511279,-0.382683432365109));
#35279=DIRECTION('',(0.,0.707106781186546,0.707106781186549));
#35280=DIRECTION('',(0.,-1.,0.));
#35281=DIRECTION('',(0.,0.,1.));
#35282=DIRECTION('center_axis',(0.,0.,1.));
#35283=DIRECTION('ref_axis',(1.,0.,0.));
#35284=DIRECTION('',(-1.,0.,0.));
#35285=DIRECTION('',(0.,-1.,0.));
#35286=DIRECTION('',(1.,0.,0.));
#35287=DIRECTION('',(0.,1.,0.));
#35288=DIRECTION('',(-1.,0.,0.));
#35289=DIRECTION('center_axis',(0.707106781186548,0.,0.707106781186548));
#35290=DIRECTION('ref_axis',(0.707106781186548,0.,-0.707106781186548));
#35291=DIRECTION('',(-0.577350269189629,-0.577350269189619,0.577350269189629));
#35292=DIRECTION('',(0.577350269189629,-0.577350269189619,-0.577350269189629));
#35293=DIRECTION('',(0.577350269189629,0.577350269189619,-0.577350269189629));
#35294=DIRECTION('',(0.,1.,0.));
#35295=DIRECTION('',(-0.577350269189616,0.577350269189646,0.577350269189616));
#35296=DIRECTION('center_axis',(0.,0.707106781186554,0.707106781186541));
#35297=DIRECTION('ref_axis',(1.,0.,0.));
#35298=DIRECTION('',(0.577350269189602,-0.577350269189633,0.577350269189643));
#35299=DIRECTION('',(-1.,0.,0.));
#35300=DIRECTION('',(0.577350269189629,0.577350269189619,-0.577350269189629));
#35301=DIRECTION('',(-0.577350269189629,0.577350269189619,-0.577350269189629));
#35302=DIRECTION('center_axis',(0.707106781186566,0.707106781186529,0.));
#35303=DIRECTION('ref_axis',(0.,0.,-1.));
#35304=DIRECTION('',(0.,0.,-1.));
#35305=DIRECTION('',(0.707106781186529,-0.707106781186566,0.));
#35306=DIRECTION('',(0.,0.,1.));
#35307=DIRECTION('center_axis',(-0.707106781186548,0.,0.707106781186548));
#35308=DIRECTION('ref_axis',(0.707106781186548,0.,0.707106781186548));
#35309=DIRECTION('',(0.577350269189629,0.577350269189619,0.577350269189629));
#35310=DIRECTION('',(-0.577350269189629,-0.577350269189619,-0.577350269189629));
#35311=DIRECTION('',(0.,-1.,0.));
#35312=DIRECTION('',(0.577350269189629,-0.577350269189619,0.577350269189629));
#35313=DIRECTION('center_axis',(0.,-0.707106781186554,0.707106781186541));
#35314=DIRECTION('ref_axis',(1.,0.,0.));
#35315=DIRECTION('',(-0.577350269189629,0.577350269189619,0.577350269189629));
#35316=DIRECTION('',(1.,0.,0.));
#35317=DIRECTION('center_axis',(-0.707106781186541,-0.707106781186554,0.));
#35318=DIRECTION('ref_axis',(0.,0.,1.));
#35319=DIRECTION('',(0.,0.,-1.));
#35320=DIRECTION('',(-0.707106781186554,0.707106781186541,0.));
#35321=DIRECTION('',(0.,0.,1.));
#35322=DIRECTION('center_axis',(0.707106781186551,0.5337451437584,0.463806124921093));
#35323=DIRECTION('ref_axis',(0.548464086412375,0.,-0.836174112201423));
#35324=DIRECTION('',(0.383127220471068,-0.840492156934371,0.383127220471115));
#35325=DIRECTION('',(-0.548464086412375,0.,0.836174112201423));
#35326=DIRECTION('',(0.,0.655920912175122,-0.75482962115391));
#35327=DIRECTION('',(-0.602464182205077,0.798145919716418,0.));
#35328=DIRECTION('',(0.,-0.655920912175122,0.75482962115391));
#35329=DIRECTION('center_axis',(0.,0.414776498746564,0.909923324290317));
#35330=DIRECTION('ref_axis',(1.,0.,0.));
#35331=DIRECTION('',(1.,0.,0.));
#35332=DIRECTION('',(-1.,0.,0.));
#35333=DIRECTION('',(0.383127220471068,0.840492156934371,-0.383127220471115));
#35334=DIRECTION('',(1.,0.,0.));
#35335=DIRECTION('',(0.,-0.909923324290317,0.414776498746564));
#35336=DIRECTION('',(1.,0.,0.));
#35337=DIRECTION('',(0.,0.909923324290317,-0.414776498746564));
#35338=DIRECTION('center_axis',(0.,0.75482962115391,0.655920912175122));
#35339=DIRECTION('ref_axis',(0.,-0.655920912175122,0.75482962115391));
#35340=DIRECTION('',(-1.,0.,0.));
#35341=DIRECTION('',(0.,0.655920912175122,-0.75482962115391));
#35342=DIRECTION('center_axis',(1.,0.,0.));
#35343=DIRECTION('ref_axis',(0.,0.,-1.));
#35344=DIRECTION('',(0.,-1.,0.));
#35345=DIRECTION('',(0.,0.923879532511279,-0.382683432365109));
#35346=DIRECTION('',(0.,-0.707106781186546,0.707106781186549));
#35347=DIRECTION('',(0.,1.,0.));
#35348=DIRECTION('',(0.,0.,1.));
#35349=DIRECTION('center_axis',(0.,0.,-1.));
#35350=DIRECTION('ref_axis',(0.,1.,0.));
#35351=DIRECTION('',(1.,0.,0.));
#35352=DIRECTION('',(0.,-1.,0.));
#35353=DIRECTION('',(-0.602464182205077,-0.798145919716418,0.));
#35354=DIRECTION('center_axis',(-0.707106781186551,0.5337451437584,0.463806124921093));
#35355=DIRECTION('ref_axis',(0.548464086412375,0.,0.836174112201423));
#35356=DIRECTION('',(0.,-0.655920912175122,0.75482962115391));
#35357=DIRECTION('',(-0.548464086412375,0.,-0.836174112201423));
#35358=DIRECTION('center_axis',(-1.,0.,0.));
#35359=DIRECTION('ref_axis',(0.,0.,1.));
#35360=DIRECTION('',(0.,0.,-1.));
#35361=DIRECTION('',(0.,0.707106781186546,-0.707106781186549));
#35362=DIRECTION('',(0.,-0.923879532511279,0.382683432365109));
#35363=DIRECTION('',(0.,1.,0.));
#35364=DIRECTION('center_axis',(-1.,0.,0.));
#35365=DIRECTION('ref_axis',(0.,0.,1.));
#35366=DIRECTION('',(0.,0.,1.));
#35367=DIRECTION('',(0.,-0.707106781186541,0.707106781186554));
#35368=DIRECTION('center_axis',(1.,0.,0.));
#35369=DIRECTION('ref_axis',(0.,0.,-1.));
#35370=DIRECTION('',(0.,0.,-1.));
#35371=DIRECTION('',(0.,0.707106781186541,-0.707106781186554));
#35372=DIRECTION('center_axis',(0.,0.,1.));
#35373=DIRECTION('ref_axis',(1.,0.,0.));
#35374=DIRECTION('',(1.,0.,0.));
#35375=DIRECTION('',(0.,1.,0.));
#35376=DIRECTION('',(-1.,0.,0.));
#35377=DIRECTION('',(0.,-1.,0.));
#35378=DIRECTION('',(1.,0.,0.));
#35379=DIRECTION('center_axis',(0.707106781186548,0.,0.707106781186548));
#35380=DIRECTION('ref_axis',(0.707106781186548,0.,-0.707106781186548));
#35381=DIRECTION('',(-0.577350269189629,-0.577350269189619,0.577350269189629));
#35382=DIRECTION('',(0.577350269189629,-0.577350269189619,-0.577350269189629));
#35383=DIRECTION('',(0.577350269189629,0.577350269189619,-0.577350269189629));
#35384=DIRECTION('',(0.,1.,0.));
#35385=DIRECTION('',(-0.577350269189616,0.577350269189646,0.577350269189616));
#35386=DIRECTION('center_axis',(0.707106781186541,-0.707106781186554,0.));
#35387=DIRECTION('ref_axis',(0.,0.,-1.));
#35388=DIRECTION('',(-0.577350269189629,-0.577350269189619,-0.577350269189629));
#35389=DIRECTION('',(0.,0.,-1.));
#35390=DIRECTION('',(-0.707106781186554,-0.707106781186541,0.));
#35391=DIRECTION('',(0.,0.,1.));
#35392=DIRECTION('center_axis',(0.,-0.707106781186554,0.707106781186541));
#35393=DIRECTION('ref_axis',(1.,0.,0.));
#35394=DIRECTION('',(0.577350269189629,0.577350269189619,0.577350269189629));
#35395=DIRECTION('',(-0.577350269189629,0.577350269189619,0.577350269189629));
#35396=DIRECTION('',(1.,0.,0.));
#35397=DIRECTION('center_axis',(-0.707106781186548,0.,0.707106781186548));
#35398=DIRECTION('ref_axis',(0.707106781186548,0.,0.707106781186548));
#35399=DIRECTION('',(-0.577350269189629,0.577350269189619,-0.577350269189629));
#35400=DIRECTION('',(-0.577350269189629,-0.577350269189619,-0.577350269189629));
#35401=DIRECTION('',(0.,-1.,0.));
#35402=DIRECTION('',(0.577350269189629,-0.577350269189619,0.577350269189629));
#35403=DIRECTION('center_axis',(-0.707106781186541,-0.707106781186554,0.));
#35404=DIRECTION('ref_axis',(0.,0.,1.));
#35405=DIRECTION('',(0.,0.,-1.));
#35406=DIRECTION('',(-0.707106781186554,0.707106781186541,0.));
#35407=DIRECTION('',(0.,0.,1.));
#35408=DIRECTION('center_axis',(0.,0.,1.));
#35409=DIRECTION('ref_axis',(-0.707106781186548,-0.707106781186548,0.));
#35410=DIRECTION('',(0.,-0.707106781186553,0.707106781186543));
#35411=DIRECTION('center_axis',(0.,0.,-1.));
#35412=DIRECTION('ref_axis',(-0.707106781186547,-0.707106781186547,0.));
#35413=DIRECTION('',(0.707106781186553,0.,-0.707106781186543));
#35414=DIRECTION('center_axis',(0.,0.,1.));
#35415=DIRECTION('ref_axis',(-0.707106781186548,-0.707106781186548,0.));
#35416=DIRECTION('center_axis',(0.,-0.707106781186543,-0.707106781186553));
#35417=DIRECTION('ref_axis',(-1.,0.,0.));
#35418=DIRECTION('',(0.,-0.707106781186553,0.707106781186543));
#35419=DIRECTION('',(-1.,0.,0.));
#35420=DIRECTION('',(1.,0.,0.));
#35421=DIRECTION('center_axis',(0.,0.,1.));
#35422=DIRECTION('ref_axis',(0.707106781186547,-0.707106781186547,0.));
#35423=DIRECTION('',(0.707106781186578,0.,0.707106781186517));
#35424=DIRECTION('center_axis',(0.,0.,-1.));
#35425=DIRECTION('ref_axis',(0.707106781186547,-0.707106781186547,0.));
#35426=DIRECTION('center_axis',(0.,0.,1.));
#35427=DIRECTION('ref_axis',(0.707106781186547,-0.707106781186547,0.));
#35428=DIRECTION('center_axis',(0.707106781186568,0.,-0.707106781186527));
#35429=DIRECTION('ref_axis',(-0.707106781186527,0.,-0.707106781186568));
#35430=DIRECTION('',(0.707106781186527,0.,0.707106781186568));
#35431=DIRECTION('',(0.,-1.,0.));
#35432=DIRECTION('',(0.,1.,0.));
#35433=DIRECTION('center_axis',(0.,0.,1.));
#35434=DIRECTION('ref_axis',(0.707106781186547,0.707106781186547,0.));
#35435=DIRECTION('',(0.,0.707106781186553,0.707106781186543));
#35436=DIRECTION('center_axis',(0.,0.,-1.));
#35437=DIRECTION('ref_axis',(0.707106781186547,0.707106781186547,0.));
#35438=DIRECTION('center_axis',(0.,0.,1.));
#35439=DIRECTION('ref_axis',(0.707106781186547,0.707106781186547,0.));
#35440=DIRECTION('center_axis',(0.,0.707106781186543,-0.707106781186553));
#35441=DIRECTION('ref_axis',(-1.,0.,0.));
#35442=DIRECTION('',(0.,0.707106781186553,0.707106781186543));
#35443=DIRECTION('',(1.,0.,0.));
#35444=DIRECTION('',(-1.,0.,0.));
#35445=DIRECTION('center_axis',(0.,0.,1.));
#35446=DIRECTION('ref_axis',(-0.707106781186548,0.707106781186548,0.));
#35447=DIRECTION('',(-0.707106781186553,0.,0.707106781186543));
#35448=DIRECTION('center_axis',(0.,0.,-1.));
#35449=DIRECTION('ref_axis',(-0.707106781186547,0.707106781186547,0.));
#35450=DIRECTION('center_axis',(0.,0.,1.));
#35451=DIRECTION('ref_axis',(-0.707106781186548,0.707106781186548,0.));
#35452=DIRECTION('center_axis',(-0.707106781186543,0.,-0.707106781186553));
#35453=DIRECTION('ref_axis',(-0.707106781186553,0.,0.707106781186543));
#35454=DIRECTION('',(0.,1.,0.));
#35455=DIRECTION('',(0.,-1.,0.));
#35456=DIRECTION('center_axis',(0.,1.,0.));
#35457=DIRECTION('ref_axis',(-1.,0.,0.));
#35458=DIRECTION('',(0.,0.,-1.));
#35459=DIRECTION('',(-1.,0.,0.));
#35460=DIRECTION('',(0.,0.,1.));
#35461=DIRECTION('center_axis',(0.,0.,1.));
#35462=DIRECTION('ref_axis',(-0.707106781186547,0.707106781186547,0.));
#35463=DIRECTION('',(0.,0.,1.));
#35464=DIRECTION('center_axis',(0.,0.,1.));
#35465=DIRECTION('ref_axis',(-0.707106781186547,0.707106781186547,0.));
#35466=DIRECTION('center_axis',(-1.,0.,0.));
#35467=DIRECTION('ref_axis',(0.,-1.,0.));
#35468=DIRECTION('',(0.,0.,-1.));
#35469=DIRECTION('',(0.,-1.,0.));
#35470=DIRECTION('center_axis',(0.,0.,1.));
#35471=DIRECTION('ref_axis',(-0.707106781186547,-0.707106781186547,0.));
#35472=DIRECTION('',(0.,0.,1.));
#35473=DIRECTION('center_axis',(0.,0.,1.));
#35474=DIRECTION('ref_axis',(-0.707106781186547,-0.707106781186547,0.));
#35475=DIRECTION('center_axis',(0.,0.,1.));
#35476=DIRECTION('ref_axis',(1.,0.,0.));
#35477=DIRECTION('center_axis',(0.,0.,-1.));
#35478=DIRECTION('ref_axis',(1.,0.,0.));
#35479=DIRECTION('center_axis',(0.,0.,-1.));
#35480=DIRECTION('ref_axis',(1.,0.,0.));
#35481=DIRECTION('center_axis',(-1.,0.,0.));
#35482=DIRECTION('ref_axis',(0.,-1.,0.));
#35483=DIRECTION('',(0.,0.,1.));
#35484=DIRECTION('',(0.,1.,0.));
#35485=DIRECTION('center_axis',(1.,0.,0.));
#35486=DIRECTION('ref_axis',(0.,1.,0.));
#35487=DIRECTION('',(0.,-1.,0.));
#35488=DIRECTION('',(0.,0.,-1.));
#35489=DIRECTION('center_axis',(-0.707106781186541,0.707106781186554,0.));
#35490=DIRECTION('ref_axis',(0.,0.,1.));
#35491=DIRECTION('',(0.577350269189629,0.577350269189619,-0.577350269189629));
#35492=DIRECTION('',(0.,0.,-1.));
#35493=DIRECTION('',(0.707106781186554,0.707106781186541,0.));
#35494=DIRECTION('center_axis',(0.,0.707106781186554,0.707106781186541));
#35495=DIRECTION('ref_axis',(1.,0.,0.));
#35496=DIRECTION('',(-1.,0.,0.));
#35497=DIRECTION('center_axis',(0.,1.,0.));
#35498=DIRECTION('ref_axis',(-1.,0.,0.));
#35499=DIRECTION('',(-1.,0.,0.));
#35500=DIRECTION('',(0.,0.,1.));
#35501=DIRECTION('',(1.,0.,0.));
#35502=DIRECTION('center_axis',(0.,1.,0.));
#35503=DIRECTION('ref_axis',(1.,0.,0.));
#35504=DIRECTION('center_axis',(0.,1.,0.));
#35505=DIRECTION('ref_axis',(1.,0.,0.));
#35506=DIRECTION('center_axis',(0.707106781186566,0.707106781186529,0.));
#35507=DIRECTION('ref_axis',(0.,0.,-1.));
#35508=DIRECTION('',(0.707106781186529,-0.707106781186566,0.));
#35509=DIRECTION('',(0.577350269189602,-0.577350269189633,0.577350269189643));
#35510=DIRECTION('center_axis',(0.,0.707106781186554,0.707106781186541));
#35511=DIRECTION('ref_axis',(1.,0.,0.));
#35512=DIRECTION('center_axis',(0.707106781186541,-0.707106781186554,0.));
#35513=DIRECTION('ref_axis',(0.,0.,-1.));
#35514=DIRECTION('',(-0.577350269189629,-0.577350269189619,-0.577350269189629));
#35515=DIRECTION('',(0.,0.,-1.));
#35516=DIRECTION('',(-0.707106781186554,-0.707106781186541,0.));
#35517=DIRECTION('',(0.,0.,1.));
#35518=DIRECTION('center_axis',(0.,-0.707106781186554,0.707106781186541));
#35519=DIRECTION('ref_axis',(1.,0.,0.));
#35520=DIRECTION('',(1.,0.,0.));
#35521=DIRECTION('center_axis',(0.,-1.,0.));
#35522=DIRECTION('ref_axis',(1.,0.,0.));
#35523=DIRECTION('',(0.,0.,-1.));
#35524=DIRECTION('',(-1.,0.,0.));
#35525=DIRECTION('center_axis',(0.,-1.,0.));
#35526=DIRECTION('ref_axis',(1.,0.,0.));
#35527=DIRECTION('center_axis',(0.,-1.,0.));
#35528=DIRECTION('ref_axis',(1.,0.,0.));
#35529=DIRECTION('center_axis',(-1.,0.,0.));
#35530=DIRECTION('ref_axis',(0.,-1.,0.));
#35531=DIRECTION('',(0.,0.,1.));
#35532=DIRECTION('',(0.,1.,0.));
#35533=DIRECTION('center_axis',(-0.707106781186541,0.707106781186554,0.));
#35534=DIRECTION('ref_axis',(0.,0.,1.));
#35535=DIRECTION('',(0.,0.,-1.));
#35536=DIRECTION('',(0.707106781186554,0.707106781186541,0.));
#35537=DIRECTION('center_axis',(1.,0.,0.));
#35538=DIRECTION('ref_axis',(0.,1.,0.));
#35539=DIRECTION('',(0.,-1.,0.));
#35540=DIRECTION('center_axis',(0.,1.,0.));
#35541=DIRECTION('ref_axis',(1.,0.,0.));
#35542=DIRECTION('center_axis',(0.,1.,0.));
#35543=DIRECTION('ref_axis',(1.,0.,0.));
#35544=DIRECTION('',(0.707106781186554,-0.707106781186541,-8.65956056235501E-17));
#35545=DIRECTION('center_axis',(0.,-1.,0.));
#35546=DIRECTION('ref_axis',(1.,0.,0.));
#35547=DIRECTION('center_axis',(0.,1.,0.));
#35548=DIRECTION('ref_axis',(1.,0.,0.));
#35549=DIRECTION('center_axis',(0.,1.,0.));
#35550=DIRECTION('ref_axis',(1.,0.,0.));
#35551=DIRECTION('',(0.,1.,0.));
#35552=DIRECTION('center_axis',(0.,1.,0.));
#35553=DIRECTION('ref_axis',(-1.,0.,0.));
#35554=DIRECTION('',(1.,0.,0.));
#35555=DIRECTION('center_axis',(0.,1.,0.));
#35556=DIRECTION('ref_axis',(1.,0.,0.));
#35557=DIRECTION('center_axis',(0.,-1.,0.));
#35558=DIRECTION('ref_axis',(1.,0.,0.));
#35559=DIRECTION('',(0.707106781186554,0.707106781186541,8.65956056235501E-17));
#35560=DIRECTION('center_axis',(0.,1.,0.));
#35561=DIRECTION('ref_axis',(1.,0.,0.));
#35562=DIRECTION('',(0.707106781186554,-0.707106781186541,-8.65956056235501E-17));
#35563=DIRECTION('center_axis',(0.,-1.,0.));
#35564=DIRECTION('ref_axis',(1.,0.,0.));
#35565=DIRECTION('center_axis',(0.,1.,0.));
#35566=DIRECTION('ref_axis',(1.,0.,0.));
#35567=DIRECTION('center_axis',(0.,1.,0.));
#35568=DIRECTION('ref_axis',(1.,0.,0.));
#35569=DIRECTION('',(0.,1.,0.));
#35570=DIRECTION('center_axis',(0.,-1.,0.));
#35571=DIRECTION('ref_axis',(1.,0.,0.));
#35572=DIRECTION('center_axis',(0.,-1.,0.));
#35573=DIRECTION('ref_axis',(1.,0.,0.));
#35574=DIRECTION('',(0.707106781186554,0.707106781186541,8.65956056235501E-17));
#35575=DIRECTION('center_axis',(0.,-1.,0.));
#35576=DIRECTION('ref_axis',(1.,0.,0.));
#35577=DIRECTION('',(-1.,0.,0.));
#35578=DIRECTION('center_axis',(0.,-1.,0.));
#35579=DIRECTION('ref_axis',(1.,0.,0.));
#35580=DIRECTION('center_axis',(0.,1.,0.));
#35581=DIRECTION('ref_axis',(1.,0.,0.));
#35582=DIRECTION('',(0.707106781186554,-0.707106781186541,-8.65956056235501E-17));
#35583=DIRECTION('center_axis',(0.,-1.,0.));
#35584=DIRECTION('ref_axis',(1.,0.,0.));
#35585=DIRECTION('center_axis',(0.,1.,0.));
#35586=DIRECTION('ref_axis',(1.,0.,0.));
#35587=DIRECTION('center_axis',(0.,1.,0.));
#35588=DIRECTION('ref_axis',(1.,0.,0.));
#35589=DIRECTION('',(0.,1.,0.));
#35590=DIRECTION('center_axis',(0.,-1.,0.));
#35591=DIRECTION('ref_axis',(1.,0.,0.));
#35592=DIRECTION('',(0.707106781186554,0.707106781186541,8.65956056235501E-17));
#35593=DIRECTION('center_axis',(0.,1.,0.));
#35594=DIRECTION('ref_axis',(1.,0.,0.));
#35595=DIRECTION('',(0.707106781186554,-0.707106781186541,-8.65956056235501E-17));
#35596=DIRECTION('center_axis',(0.,-1.,0.));
#35597=DIRECTION('ref_axis',(1.,0.,0.));
#35598=DIRECTION('center_axis',(0.,1.,0.));
#35599=DIRECTION('ref_axis',(1.,0.,0.));
#35600=DIRECTION('center_axis',(0.,1.,0.));
#35601=DIRECTION('ref_axis',(1.,0.,0.));
#35602=DIRECTION('',(0.,1.,0.));
#35603=DIRECTION('center_axis',(0.,-1.,0.));
#35604=DIRECTION('ref_axis',(1.,0.,0.));
#35605=DIRECTION('',(0.707106781186554,0.707106781186541,8.65956056235501E-17));
#35606=DIRECTION('center_axis',(0.,0.,-1.));
#35607=DIRECTION('ref_axis',(1.,0.,0.));
#35608=DIRECTION('',(0.707106781186553,-8.65956056235499E-17,0.707106781186543));
#35609=DIRECTION('center_axis',(0.,0.,1.));
#35610=DIRECTION('ref_axis',(1.,0.,0.));
#35611=DIRECTION('center_axis',(0.,0.,1.));
#35612=DIRECTION('ref_axis',(1.,0.,0.));
#35613=DIRECTION('',(0.,0.,1.));
#35614=DIRECTION('center_axis',(0.,0.,-1.));
#35615=DIRECTION('ref_axis',(1.,0.,0.));
#35616=DIRECTION('center_axis',(0.,0.,-1.));
#35617=DIRECTION('ref_axis',(1.,0.,0.));
#35618=DIRECTION('',(0.707106781186553,-8.65956056235499E-17,0.707106781186543));
#35619=DIRECTION('center_axis',(0.,0.,1.));
#35620=DIRECTION('ref_axis',(1.,0.,0.));
#35621=DIRECTION('center_axis',(0.,0.,1.));
#35622=DIRECTION('ref_axis',(1.,0.,0.));
#35623=DIRECTION('',(0.,0.,1.));
#35624=DIRECTION('center_axis',(0.,0.,-1.));
#35625=DIRECTION('ref_axis',(1.,0.,0.));
#35626=DIRECTION('center_axis',(0.,-0.382683432365109,0.923879532511279));
#35627=DIRECTION('ref_axis',(1.,0.,0.));
#35628=DIRECTION('',(-1.,0.,0.));
#35629=DIRECTION('',(0.,-0.92387953251128,-0.382683432365107));
#35630=DIRECTION('',(1.,0.,0.));
#35631=DIRECTION('center_axis',(0.,0.,-1.));
#35632=DIRECTION('ref_axis',(-0.707106781186547,-0.707106781186547,0.));
#35633=DIRECTION('',(-0.923879532511284,0.,-0.382683432365098));
#35634=DIRECTION('center_axis',(0.,0.,1.));
#35635=DIRECTION('ref_axis',(-0.707106781186548,-0.707106781186548,0.));
#35636=DIRECTION('center_axis',(0.,0.,-1.));
#35637=DIRECTION('ref_axis',(-0.707106781186547,-0.707106781186547,0.));
#35638=DIRECTION('center_axis',(-0.382683432365094,0.,0.923879532511285));
#35639=DIRECTION('ref_axis',(0.923879532511285,0.,0.382683432365094));
#35640=DIRECTION('',(-0.923879532511286,0.,-0.382683432365091));
#35641=DIRECTION('',(0.,-1.,0.));
#35642=DIRECTION('',(0.,1.,0.));
#35643=DIRECTION('center_axis',(0.,0.,-1.));
#35644=DIRECTION('ref_axis',(-0.707106781186547,0.707106781186547,0.));
#35645=DIRECTION('',(0.,0.923879532511284,-0.382683432365098));
#35646=DIRECTION('center_axis',(0.,0.,1.));
#35647=DIRECTION('ref_axis',(-0.707106781186548,0.707106781186548,0.));
#35648=DIRECTION('center_axis',(0.,0.,-1.));
#35649=DIRECTION('ref_axis',(-0.707106781186547,0.707106781186547,0.));
#35650=DIRECTION('center_axis',(0.,0.382683432365109,0.923879532511279));
#35651=DIRECTION('ref_axis',(1.,0.,0.));
#35652=DIRECTION('',(-1.,0.,0.));
#35653=DIRECTION('',(1.,0.,0.));
#35654=DIRECTION('center_axis',(0.,0.,1.));
#35655=DIRECTION('ref_axis',(1.,0.,0.));
#35656=DIRECTION('',(0.,-1.,0.));
#35657=DIRECTION('',(-1.,0.,0.));
#35658=DIRECTION('center_axis',(0.,0.,-1.));
#35659=DIRECTION('ref_axis',(0.707106781186548,-0.707106781186548,0.));
#35660=DIRECTION('',(0.,-1.,0.));
#35661=DIRECTION('center_axis',(0.,0.,-1.));
#35662=DIRECTION('ref_axis',(0.707106781186548,0.707106781186548,0.));
#35663=DIRECTION('',(1.,0.,0.));
#35664=DIRECTION('center_axis',(0.,0.,1.));
#35665=DIRECTION('ref_axis',(1.,0.,0.));
#35666=DIRECTION('center_axis',(0.,0.,1.));
#35667=DIRECTION('ref_axis',(1.,0.,0.));
#35668=DIRECTION('center_axis',(0.,0.382683432365109,0.923879532511279));
#35669=DIRECTION('ref_axis',(1.,0.,0.));
#35670=DIRECTION('',(0.,0.923879532511282,-0.382683432365102));
#35671=DIRECTION('',(-1.,0.,0.));
#35672=DIRECTION('center_axis',(0.,0.,-1.));
#35673=DIRECTION('ref_axis',(0.707106781186547,0.707106781186548,0.));
#35674=DIRECTION('',(0.923879532511287,1.92271478790291E-14,-0.38268343236509));
#35675=DIRECTION('center_axis',(0.,0.,1.));
#35676=DIRECTION('ref_axis',(0.707106781186546,0.707106781186549,0.));
#35677=DIRECTION('center_axis',(0.382683432365089,0.,0.923879532511287));
#35678=DIRECTION('ref_axis',(0.923879532511287,0.,-0.382683432365089));
#35679=DIRECTION('',(0.923879532511287,0.,-0.38268343236509));
#35680=DIRECTION('',(0.,1.,0.));
#35681=DIRECTION('center_axis',(0.,0.,-1.));
#35682=DIRECTION('ref_axis',(0.707106781186547,-0.707106781186548,0.));
#35683=DIRECTION('',(0.,-0.923879532511287,-0.38268343236509));
#35684=DIRECTION('center_axis',(0.,0.,1.));
#35685=DIRECTION('ref_axis',(0.707106781186546,-0.707106781186549,0.));
#35686=DIRECTION('center_axis',(0.,-0.382683432365109,0.923879532511279));
#35687=DIRECTION('ref_axis',(1.,0.,0.));
#35688=DIRECTION('',(0.,0.923879532511279,0.382683432365109));
#35689=DIRECTION('',(1.,0.,0.));
#35690=DIRECTION('center_axis',(0.,0.,1.));
#35691=DIRECTION('ref_axis',(1.,0.,0.));
#35692=DIRECTION('',(0.707106781186553,8.65956056235499E-17,-0.707106781186542));
#35693=DIRECTION('center_axis',(0.,0.,1.));
#35694=DIRECTION('ref_axis',(1.,0.,0.));
#35695=DIRECTION('',(0.707106781186553,8.65956056235499E-17,-0.707106781186542));
#35696=DIRECTION('center_axis',(0.,-0.75482962115391,0.655920912175122));
#35697=DIRECTION('ref_axis',(0.,-0.655920912175122,-0.75482962115391));
#35698=DIRECTION('',(-1.,0.,0.));
#35699=DIRECTION('center_axis',(0.,0.,-1.));
#35700=DIRECTION('ref_axis',(0.,1.,0.));
#35701=DIRECTION('',(-1.,0.,0.));
#35702=DIRECTION('',(0.,1.,0.));
#35703=DIRECTION('center_axis',(1.,0.,0.));
#35704=DIRECTION('ref_axis',(0.,0.,-1.));
#35705=DIRECTION('',(0.,-0.707106781186546,-0.707106781186549));
#35706=DIRECTION('center_axis',(0.,0.,-1.));
#35707=DIRECTION('ref_axis',(-0.707106781186548,-0.707106781186548,0.));
#35708=DIRECTION('',(-0.707106781186553,0.,-0.707106781186542));
#35709=DIRECTION('',(0.,0.707106781186553,0.707106781186542));
#35710=DIRECTION('center_axis',(-0.707106781186549,0.,0.707106781186546));
#35711=DIRECTION('ref_axis',(0.707106781186546,0.,0.707106781186549));
#35712=DIRECTION('',(-0.707106781186546,0.,-0.707106781186549));
#35713=DIRECTION('center_axis',(0.,0.,-1.));
#35714=DIRECTION('ref_axis',(-0.707106781186548,0.707106781186548,0.));
#35715=DIRECTION('',(0.,0.707106781186553,-0.707106781186542));
#35716=DIRECTION('center_axis',(0.,0.707106781186549,0.707106781186546));
#35717=DIRECTION('ref_axis',(1.,0.,0.));
#35718=DIRECTION('',(0.,0.707106781186546,-0.707106781186549));
#35719=DIRECTION('center_axis',(0.,0.,-1.));
#35720=DIRECTION('ref_axis',(0.707106781186548,0.707106781186548,0.));
#35721=DIRECTION('',(0.707106781186553,0.,-0.707106781186542));
#35722=DIRECTION('center_axis',(0.,0.,1.));
#35723=DIRECTION('ref_axis',(0.707106781186547,0.707106781186547,0.));
#35724=DIRECTION('center_axis',(0.707106781186542,0.,0.707106781186553));
#35725=DIRECTION('ref_axis',(0.707106781186553,0.,-0.707106781186542));
#35726=DIRECTION('',(0.707106781186553,0.,-0.707106781186542));
#35727=DIRECTION('',(0.,1.,0.));
#35728=DIRECTION('center_axis',(0.,0.,-1.));
#35729=DIRECTION('ref_axis',(0.707106781186548,-0.707106781186548,0.));
#35730=DIRECTION('',(0.,-0.707106781186553,-0.707106781186542));
#35731=DIRECTION('center_axis',(0.,0.,1.));
#35732=DIRECTION('ref_axis',(0.707106781186547,-0.707106781186547,0.));
#35733=DIRECTION('center_axis',(0.,-0.707106781186549,0.707106781186546));
#35734=DIRECTION('ref_axis',(1.,0.,0.));
#35735=DIRECTION('',(1.,0.,0.));
#35736=DIRECTION('center_axis',(1.,0.,0.));
#35737=DIRECTION('ref_axis',(0.,1.,0.));
#35738=DIRECTION('',(0.,0.,-1.));
#35739=DIRECTION('',(0.,0.,1.));
#35740=DIRECTION('center_axis',(0.,0.,1.));
#35741=DIRECTION('ref_axis',(0.707106781186547,-0.707106781186547,0.));
#35742=DIRECTION('',(0.,0.,-1.));
#35743=DIRECTION('center_axis',(0.,-1.,0.));
#35744=DIRECTION('ref_axis',(1.,0.,0.));
#35745=DIRECTION('center_axis',(0.,0.,1.));
#35746=DIRECTION('ref_axis',(0.707106781186547,0.707106781186547,0.));
#50002=CARTESIAN_POINT('',(0.,0.,0.));
#50003=CARTESIAN_POINT('Origin',(30.75,9.51646399110419,18.4280916795304));
#50004=CARTESIAN_POINT('',(30.8,4.8,24.1560450044147));
#50005=CARTESIAN_POINT('',(30.7,4.8,24.));
#50006=CARTESIAN_POINT('',(24.6978189959578,4.8,14.6338963872653));
#50007=CARTESIAN_POINT('',(30.7,24.,1.));
#50008=CARTESIAN_POINT('',(30.7,9.4780802994519,18.3960496412816));
#50009=CARTESIAN_POINT('',(30.8,24.1302636558592,1.));
#50010=CARTESIAN_POINT('',(21.980595587918,12.6417850436725,0.999999999999998));
#50011=CARTESIAN_POINT('',(30.8,9.55484768275647,18.4601337177793));
#50012=CARTESIAN_POINT('Origin',(30.,4.8,24.));
#50013=CARTESIAN_POINT('',(29.3,4.8,24.));
#50014=CARTESIAN_POINT('',(32.,4.8,24.));
#50015=CARTESIAN_POINT('',(29.3,24.,1.));
#50016=CARTESIAN_POINT('',(29.3,9.4780802994519,18.3960496412816));
#50017=CARTESIAN_POINT('',(31.875,24.,1.));
#50018=CARTESIAN_POINT('Origin',(29.25,9.51646399110419,18.4280916795304));
#50019=CARTESIAN_POINT('',(29.2,24.1302636558592,1.));
#50020=CARTESIAN_POINT('',(39.4099093747916,10.8304624443433,1.));
#50021=CARTESIAN_POINT('',(29.2,4.8,24.1560450044147));
#50022=CARTESIAN_POINT('',(36.4666627932199,4.8,12.8167807279347));
#50023=CARTESIAN_POINT('',(29.2,9.55484768275647,18.4601337177793));
#50024=CARTESIAN_POINT('Origin',(30.75,-19.1164639911042,6.92809167953045));
#50025=CARTESIAN_POINT('',(30.8,-24.1302636558592,1.));
#50026=CARTESIAN_POINT('',(30.7,-24.,1.));
#50027=CARTESIAN_POINT('',(24.2990885150594,-15.6619386914043,1.));
#50028=CARTESIAN_POINT('',(30.7,-4.8,24.));
#50029=CARTESIAN_POINT('',(30.7,-19.0780802994519,6.89604964128158));
#50030=CARTESIAN_POINT('',(30.8,-4.8,24.1560450044147));
#50031=CARTESIAN_POINT('',(20.9212334464924,-4.8,8.74072329987777));
#50032=CARTESIAN_POINT('',(30.8,-19.1548476827565,6.96013371777932));
#50033=CARTESIAN_POINT('Origin',(30.,-24.,1.));
#50034=CARTESIAN_POINT('',(29.3,-24.,1.));
#50035=CARTESIAN_POINT('',(31.875,-24.,1.));
#50036=CARTESIAN_POINT('',(29.3,-4.8,24.));
#50037=CARTESIAN_POINT('',(29.3,-19.0780802994519,6.89604964128158));
#50038=CARTESIAN_POINT('',(28.,-4.8,24.));
#50039=CARTESIAN_POINT('Origin',(29.25,-19.1164639911042,6.92809167953045));
#50040=CARTESIAN_POINT('',(29.2,-4.8,24.1560450044147));
#50041=CARTESIAN_POINT('',(37.9142847643299,-4.8,10.5578389592083));
#50042=CARTESIAN_POINT('',(29.2,-24.1302636558592,1.));
#50043=CARTESIAN_POINT('',(37.0914164476502,-13.850616092075,0.999999999999999));
#50044=CARTESIAN_POINT('',(29.2,-19.1548476827565,6.96013371777932));
#50045=CARTESIAN_POINT('Origin',(30.75,-11.0622585189423,22.7172039543912));
#50046=CARTESIAN_POINT('',(30.7,-30.,1.));
#50047=CARTESIAN_POINT('',(30.8,-29.8675197724128,1.));
#50048=CARTESIAN_POINT('',(35.1351844799295,-24.124257507079,1.));
#50049=CARTESIAN_POINT('',(30.8,-4.8,29.847542595237));
#50050=CARTESIAN_POINT('',(30.8,-11.0245170378846,22.6844079087825));
#50051=CARTESIAN_POINT('',(30.7298992862524,-4.8,29.954416324137));
#50052=CARTESIAN_POINT('',(38.3204633389669,-4.8,18.382039362495));
#50053=CARTESIAN_POINT('',(30.7,-4.86559209121751,29.9245170378846));
#50054=CARTESIAN_POINT('',(29.1417160738286,-8.28410518097803,28.3662331117132));
#50055=CARTESIAN_POINT('',(30.7,-11.1,22.75));
#50056=CARTESIAN_POINT('Origin',(30.,-4.78279604560876,29.9622585189423));
#50057=CARTESIAN_POINT('',(30.8,-4.8,29.954416324137));
#50058=CARTESIAN_POINT('',(28.,-4.8,29.954416324137));
#50059=CARTESIAN_POINT('',(30.8,-4.7,30.));
#50060=CARTESIAN_POINT('',(30.8,-12.7352042956433,26.3372585189423));
#50061=CARTESIAN_POINT('',(29.2,-4.7,30.));
#50062=CARTESIAN_POINT('',(30.,-4.7,30.));
#50063=CARTESIAN_POINT('',(29.2,-4.8,29.954416324137));
#50064=CARTESIAN_POINT('',(29.2,-12.7352042956433,26.3372585189423));
#50065=CARTESIAN_POINT('',(29.2701007137476,-4.8,29.954416324137));
#50066=CARTESIAN_POINT('',(28.,-4.8,29.954416324137));
#50067=CARTESIAN_POINT('',(29.3,-4.86559209121751,29.9245170378846));
#50068=CARTESIAN_POINT('',(30.8582839261714,-8.28410518097803,28.3662331117132));
#50069=CARTESIAN_POINT('',(30.,-4.86559209121751,29.9245170378846));
#50070=CARTESIAN_POINT('Origin',(30.8,-17.4,15.5));
#50071=CARTESIAN_POINT('',(30.8,-4.8,29.9));
#50072=CARTESIAN_POINT('',(30.8,-4.8,8.25));
#50073=CARTESIAN_POINT('',(30.8,-11.5249999999999,23.1749999999999));
#50074=CARTESIAN_POINT('Origin',(29.25,-11.0622585189423,22.7172039543912));
#50075=CARTESIAN_POINT('',(29.2,-4.8,29.847542595237));
#50076=CARTESIAN_POINT('',(20.4762852446965,-4.8,16.547593480374));
#50077=CARTESIAN_POINT('',(29.2,-29.8675197724128,1.));
#50078=CARTESIAN_POINT('',(29.2,-11.0245170378846,22.6844079087825));
#50079=CARTESIAN_POINT('',(29.3,-30.,1.));
#50080=CARTESIAN_POINT('',(24.8648155200705,-24.124257507079,1.));
#50081=CARTESIAN_POINT('',(29.3,-11.1,22.75));
#50082=CARTESIAN_POINT('Origin',(29.2,-17.4,15.5));
#50083=CARTESIAN_POINT('',(29.2,-4.8,29.9));
#50084=CARTESIAN_POINT('',(29.2,-4.8,8.25));
#50085=CARTESIAN_POINT('',(29.2,-11.5249999999999,23.1749999999999));
#50086=CARTESIAN_POINT('Origin',(29.2,-17.4,15.5));
#50087=CARTESIAN_POINT('',(29.2,-29.7,1.));
#50088=CARTESIAN_POINT('',(29.2,-8.7,1.));
#50089=CARTESIAN_POINT('',(29.2,-29.8707106781187,0.929289321881342));
#50090=CARTESIAN_POINT('',(29.2,-21.9300622355798,4.21841360081793));
#50091=CARTESIAN_POINT('',(29.2,-29.8,1.));
#50092=CARTESIAN_POINT('',(29.2,-23.125,7.67500000000001));
#50093=CARTESIAN_POINT('',(29.2,-24.,1.));
#50094=CARTESIAN_POINT('',(29.2,-4.8,8.25));
#50095=CARTESIAN_POINT('Origin',(30.,-4.4,30.));
#50096=CARTESIAN_POINT('',(33.9,-4.7,30.));
#50097=CARTESIAN_POINT('',(28.,-4.7,30.));
#50098=CARTESIAN_POINT('',(33.9,-4.1,30.));
#50099=CARTESIAN_POINT('',(33.9,-4.6,30.));
#50100=CARTESIAN_POINT('',(26.1,-4.1,30.));
#50101=CARTESIAN_POINT('',(32.,-4.1,30.));
#50102=CARTESIAN_POINT('',(26.1,-4.7,30.));
#50103=CARTESIAN_POINT('',(26.1,-4.2,30.));
#50104=CARTESIAN_POINT('',(28.,-4.7,30.));
#50105=CARTESIAN_POINT('Origin',(33.95,-4.6,29.95));
#50106=CARTESIAN_POINT('',(33.95,-4.05,29.95));
#50107=CARTESIAN_POINT('',(33.5333333333333,-4.46666666666666,30.3666666666667));
#50108=CARTESIAN_POINT('',(33.95,-4.75,29.95));
#50109=CARTESIAN_POINT('',(32.9333333333333,-3.73333333333334,30.9666666666667));
#50110=CARTESIAN_POINT('',(34.,-4.7,29.9));
#50111=CARTESIAN_POINT('',(38.8000000000001,0.0999999999999677,25.0999999999999));
#50112=CARTESIAN_POINT('',(34.,-4.1,29.9));
#50113=CARTESIAN_POINT('',(34.,-4.6,29.9));
#50114=CARTESIAN_POINT('',(38.8666666666665,-8.96666666666676,25.0333333333335));
#50115=CARTESIAN_POINT('Origin',(32.,-4.05,29.95));
#50116=CARTESIAN_POINT('',(33.9,-4.,29.9));
#50117=CARTESIAN_POINT('',(33.9,-4.,29.9));
#50118=CARTESIAN_POINT('',(26.1,-4.,29.9));
#50119=CARTESIAN_POINT('',(32.,-4.,29.9));
#50120=CARTESIAN_POINT('',(26.05,-4.05,29.95));
#50121=CARTESIAN_POINT('',(26.,-4.1,30.));
#50122=CARTESIAN_POINT('',(27.0666666666667,-5.06666666666666,30.9666666666667));
#50123=CARTESIAN_POINT('Origin',(33.95,-4.05,1.));
#50124=CARTESIAN_POINT('',(34.,-4.1,1.));
#50125=CARTESIAN_POINT('',(34.,-4.1,1.));
#50126=CARTESIAN_POINT('',(33.9,-4.,1.));
#50127=CARTESIAN_POINT('',(32.8875,-2.98749999999995,1.));
#50128=CARTESIAN_POINT('',(33.9,-4.,1.));
#50129=CARTESIAN_POINT('Origin',(26.05,-4.2,29.95));
#50130=CARTESIAN_POINT('',(26.05,-4.75,29.95));
#50131=CARTESIAN_POINT('',(26.4666666666667,-4.33333333333334,30.3666666666667));
#50132=CARTESIAN_POINT('',(26.,-4.1,29.9));
#50133=CARTESIAN_POINT('',(21.1999999999999,-8.89999999999997,25.0999999999999));
#50134=CARTESIAN_POINT('',(26.,-4.7,29.9));
#50135=CARTESIAN_POINT('',(26.,-4.2,29.9));
#50136=CARTESIAN_POINT('',(21.1333333333333,0.166666666666632,25.0333333333333));
#50137=CARTESIAN_POINT('Origin',(28.,-4.75,29.95));
#50138=CARTESIAN_POINT('',(26.1,-4.8,29.9));
#50139=CARTESIAN_POINT('',(26.1,-4.8,29.9));
#50140=CARTESIAN_POINT('',(28.,-4.8,29.9));
#50141=CARTESIAN_POINT('Origin',(26.05,-4.75,1.));
#50142=CARTESIAN_POINT('',(26.,-4.7,1.));
#50143=CARTESIAN_POINT('',(26.,-4.7,1.));
#50144=CARTESIAN_POINT('',(26.1,-4.8,1.));
#50145=CARTESIAN_POINT('',(26.7875,-5.48750000000002,1.));
#50146=CARTESIAN_POINT('',(26.1,-4.8,1.));
#50147=CARTESIAN_POINT('Origin',(30.75,23.6622585189423,8.21720395439124));
#50148=CARTESIAN_POINT('',(30.7,4.86559209121751,29.9245170378846));
#50149=CARTESIAN_POINT('',(30.7298992862524,4.8,29.954416324137));
#50150=CARTESIAN_POINT('',(26.0488170169426,15.0692075193245,25.2733340548267));
#50151=CARTESIAN_POINT('',(30.8,4.8,29.847542595237));
#50152=CARTESIAN_POINT('',(42.8486479166477,4.8,11.4784866724842));
#50153=CARTESIAN_POINT('',(30.8,29.8675197724128,1.));
#50154=CARTESIAN_POINT('',(30.8,23.6245170378846,8.18440790878249));
#50155=CARTESIAN_POINT('',(30.7,30.,1.));
#50156=CARTESIAN_POINT('',(33.548365194882,26.2264793073069,1.));
#50157=CARTESIAN_POINT('',(30.7,23.7,8.25));
#50158=CARTESIAN_POINT('Origin',(30.,4.78279604560876,29.9622585189423));
#50159=CARTESIAN_POINT('',(30.8,4.8,29.954416324137));
#50160=CARTESIAN_POINT('',(32.,4.8,29.954416324137));
#50161=CARTESIAN_POINT('',(29.3,4.86559209121751,29.9245170378846));
#50162=CARTESIAN_POINT('',(30.,4.86559209121751,29.9245170378846));
#50163=CARTESIAN_POINT('',(29.2701007137476,4.8,29.954416324137));
#50164=CARTESIAN_POINT('',(33.9511829830574,15.0692075193245,25.2733340548267));
#50165=CARTESIAN_POINT('',(29.2,4.8,29.954416324137));
#50166=CARTESIAN_POINT('',(32.,4.8,29.954416324137));
#50167=CARTESIAN_POINT('',(29.2,4.7,30.));
#50168=CARTESIAN_POINT('',(29.2,12.7352042956433,26.3372585189421));
#50169=CARTESIAN_POINT('',(30.8,4.7,30.));
#50170=CARTESIAN_POINT('',(30.,4.7,30.));
#50171=CARTESIAN_POINT('',(30.8,12.7352042956433,26.3372585189421));
#50172=CARTESIAN_POINT('Origin',(30.,30.,1.));
#50173=CARTESIAN_POINT('',(29.3,30.,1.));
#50174=CARTESIAN_POINT('',(30.,30.,1.));
#50175=CARTESIAN_POINT('',(29.3,23.7,8.25));
#50176=CARTESIAN_POINT('Origin',(30.8,17.4,15.5));
#50177=CARTESIAN_POINT('',(30.8,29.7,1.));
#50178=CARTESIAN_POINT('',(30.8,8.7,1.));
#50179=CARTESIAN_POINT('',(30.8,29.8707106781187,0.929289321881342));
#50180=CARTESIAN_POINT('',(30.8,21.9300622355798,4.21841360081793));
#50181=CARTESIAN_POINT('',(30.8,29.8,1.));
#50182=CARTESIAN_POINT('',(30.8,23.125,7.67500000000001));
#50183=CARTESIAN_POINT('',(30.8,24.,1.));
#50184=CARTESIAN_POINT('',(30.8,4.8,8.25));
#50185=CARTESIAN_POINT('Origin',(30.,24.,1.));
#50186=CARTESIAN_POINT('',(29.2,29.8,1.));
#50187=CARTESIAN_POINT('',(38.125,29.8,1.));
#50188=CARTESIAN_POINT('',(29.2,29.8675197724128,1.));
#50189=CARTESIAN_POINT('',(29.2,24.,1.));
#50190=CARTESIAN_POINT('',(26.451634805118,26.2264793073069,1.));
#50191=CARTESIAN_POINT('Origin',(29.25,23.6622585189423,8.21720395439124));
#50192=CARTESIAN_POINT('',(29.2,4.8,29.847542595237));
#50193=CARTESIAN_POINT('',(29.2,23.6245170378846,8.18440790878249));
#50194=CARTESIAN_POINT('',(18.3546034996889,4.8,13.3129325546051));
#50195=CARTESIAN_POINT('Origin',(29.2,17.4,15.5));
#50196=CARTESIAN_POINT('',(29.2,4.8,8.25));
#50197=CARTESIAN_POINT('',(29.2,29.8707106781187,0.929289321881342));
#50198=CARTESIAN_POINT('',(29.2,23.125,7.67500000000001));
#50199=CARTESIAN_POINT('',(29.2,29.7,1.));
#50200=CARTESIAN_POINT('',(29.2,21.9300622355798,4.21841360081793));
#50201=CARTESIAN_POINT('',(29.2,8.7,1.));
#50202=CARTESIAN_POINT('Origin',(29.2,17.4,15.5));
#50203=CARTESIAN_POINT('',(29.2,4.8,29.9));
#50204=CARTESIAN_POINT('',(29.2,4.8,8.25));
#50205=CARTESIAN_POINT('',(29.2,11.5249999999999,23.1749999999999));
#50206=CARTESIAN_POINT('Origin',(30.8,17.4,15.5));
#50207=CARTESIAN_POINT('',(30.8,4.8,29.9));
#50208=CARTESIAN_POINT('',(30.8,4.8,8.25));
#50209=CARTESIAN_POINT('',(30.8,11.5249999999999,23.1749999999999));
#50210=CARTESIAN_POINT('Origin',(30.,4.4,30.));
#50211=CARTESIAN_POINT('',(26.1,4.7,30.));
#50212=CARTESIAN_POINT('',(32.,4.7,30.));
#50213=CARTESIAN_POINT('',(26.1,4.1,30.));
#50214=CARTESIAN_POINT('',(26.1,4.6,30.));
#50215=CARTESIAN_POINT('',(33.9,4.1,30.));
#50216=CARTESIAN_POINT('',(28.,4.1,30.));
#50217=CARTESIAN_POINT('',(33.9,4.7,30.));
#50218=CARTESIAN_POINT('',(33.9,4.2,30.));
#50219=CARTESIAN_POINT('',(32.,4.7,30.));
#50220=CARTESIAN_POINT('Origin',(33.95,4.2,29.95));
#50221=CARTESIAN_POINT('',(33.95,4.75,29.95));
#50222=CARTESIAN_POINT('',(33.5333333333333,4.33333333333334,30.3666666666667));
#50223=CARTESIAN_POINT('',(33.95,4.05,29.95));
#50224=CARTESIAN_POINT('',(32.9333333333333,5.06666666666666,30.9666666666667));
#50225=CARTESIAN_POINT('',(34.,4.1,29.9));
#50226=CARTESIAN_POINT('',(38.8000000000001,8.89999999999997,25.0999999999999));
#50227=CARTESIAN_POINT('',(34.,4.7,29.9));
#50228=CARTESIAN_POINT('',(34.,4.2,29.9));
#50229=CARTESIAN_POINT('',(38.8666666666665,-0.166666666666758,25.0333333333335));
#50230=CARTESIAN_POINT('Origin',(33.95,4.05,1.));
#50231=CARTESIAN_POINT('',(33.9,4.,29.9));
#50232=CARTESIAN_POINT('',(34.,4.1,30.));
#50233=CARTESIAN_POINT('',(33.9,4.,1.));
#50234=CARTESIAN_POINT('',(33.9,4.,1.));
#50235=CARTESIAN_POINT('',(34.,4.1,1.));
#50236=CARTESIAN_POINT('',(32.8875,2.98750000000002,1.));
#50237=CARTESIAN_POINT('',(34.,4.1,1.));
#50238=CARTESIAN_POINT('Origin',(28.,4.05,29.95));
#50239=CARTESIAN_POINT('',(26.05,4.05,29.95));
#50240=CARTESIAN_POINT('',(26.4666666666667,4.46666666666666,30.3666666666667));
#50241=CARTESIAN_POINT('',(26.1,4.,29.9));
#50242=CARTESIAN_POINT('',(26.1,4.,29.9));
#50243=CARTESIAN_POINT('',(28.,4.,29.9));
#50244=CARTESIAN_POINT('Origin',(26.05,4.6,29.95));
#50245=CARTESIAN_POINT('',(26.05,4.75,29.95));
#50246=CARTESIAN_POINT('',(27.0666666666667,3.73333333333334,30.9666666666667));
#50247=CARTESIAN_POINT('',(26.,4.7,29.9));
#50248=CARTESIAN_POINT('',(21.1999999999999,-0.0999999999999677,25.0999999999999));
#50249=CARTESIAN_POINT('',(26.,4.1,29.9));
#50250=CARTESIAN_POINT('',(26.,4.6,29.9));
#50251=CARTESIAN_POINT('',(21.1333333333333,8.96666666666663,25.0333333333333));
#50252=CARTESIAN_POINT('Origin',(26.05,4.05,1.));
#50253=CARTESIAN_POINT('',(26.,4.1,1.));
#50254=CARTESIAN_POINT('',(26.,4.1,1.));
#50255=CARTESIAN_POINT('',(26.1,4.,1.));
#50256=CARTESIAN_POINT('',(28.9875,1.11250000000002,1.));
#50257=CARTESIAN_POINT('',(26.1,4.,1.));
#50258=CARTESIAN_POINT('Origin',(26.5,-28.5,0.05));
#50259=CARTESIAN_POINT('',(26.5,-29.9,0.));
#50260=CARTESIAN_POINT('',(26.5,-30.,0.1));
#50261=CARTESIAN_POINT('',(26.5,-29.9,0.));
#50262=CARTESIAN_POINT('',(25.,-28.5,0.1));
#50263=CARTESIAN_POINT('Origin',(26.5,-28.5,0.1));
#50264=CARTESIAN_POINT('',(25.1,-28.5,0.));
#50265=CARTESIAN_POINT('',(25.,-28.5,0.1));
#50266=CARTESIAN_POINT('Origin',(26.5,-28.5,0.));
#50267=CARTESIAN_POINT('Origin',(29.375,-29.95,0.05));
#50268=CARTESIAN_POINT('',(41.,-29.9,0.));
#50269=CARTESIAN_POINT('',(41.,-30.,0.1));
#50270=CARTESIAN_POINT('',(41.,-29.9,0.));
#50271=CARTESIAN_POINT('',(29.375,-30.,0.1));
#50272=CARTESIAN_POINT('',(29.375,-29.9,0.));
#50273=CARTESIAN_POINT('Origin',(41.,-28.5,0.05));
#50274=CARTESIAN_POINT('',(42.4,-28.5,0.));
#50275=CARTESIAN_POINT('',(42.5,-28.5,0.1));
#50276=CARTESIAN_POINT('',(42.4,-28.5,0.));
#50277=CARTESIAN_POINT('Origin',(41.,-28.5,0.1));
#50278=CARTESIAN_POINT('Origin',(41.,-28.5,0.));
#50279=CARTESIAN_POINT('Origin',(42.45,-15.,0.05));
#50280=CARTESIAN_POINT('',(42.4,28.5,0.));
#50281=CARTESIAN_POINT('',(42.5,28.5,0.1));
#50282=CARTESIAN_POINT('',(42.4,28.5,0.));
#50283=CARTESIAN_POINT('',(42.5,-15.,0.1));
#50284=CARTESIAN_POINT('',(42.4,-15.,0.));
#50285=CARTESIAN_POINT('Origin',(41.,28.5,0.05));
#50286=CARTESIAN_POINT('',(41.,29.9,0.));
#50287=CARTESIAN_POINT('',(41.,30.,0.1));
#50288=CARTESIAN_POINT('',(41.,29.9,0.));
#50289=CARTESIAN_POINT('Origin',(41.,28.5,0.1));
#50290=CARTESIAN_POINT('Origin',(41.,28.5,0.));
#50291=CARTESIAN_POINT('Origin',(38.125,29.95,0.05));
#50292=CARTESIAN_POINT('',(26.5,29.9,0.));
#50293=CARTESIAN_POINT('',(26.5,30.,0.1));
#50294=CARTESIAN_POINT('',(26.5,29.9,0.));
#50295=CARTESIAN_POINT('',(38.125,30.,0.1));
#50296=CARTESIAN_POINT('',(38.125,29.9,0.));
#50297=CARTESIAN_POINT('Origin',(26.5,28.5,0.05));
#50298=CARTESIAN_POINT('',(25.1,28.5,0.));
#50299=CARTESIAN_POINT('',(25.,28.5,0.1));
#50300=CARTESIAN_POINT('',(25.1,28.5,0.));
#50301=CARTESIAN_POINT('Origin',(26.5,28.5,0.1));
#50302=CARTESIAN_POINT('Origin',(26.5,28.5,0.));
#50303=CARTESIAN_POINT('Origin',(25.05,15.,0.05));
#50304=CARTESIAN_POINT('',(25.,15.,0.1));
#50305=CARTESIAN_POINT('',(25.1,15.,0.));
#50306=CARTESIAN_POINT('Origin',(42.5,30.,0.));
#50307=CARTESIAN_POINT('',(26.5,30.,0.8));
#50308=CARTESIAN_POINT('',(26.5,30.,0.));
#50309=CARTESIAN_POINT('',(41.,30.,0.8));
#50310=CARTESIAN_POINT('',(38.125,30.,0.8));
#50311=CARTESIAN_POINT('',(41.,30.,0.));
#50312=CARTESIAN_POINT('Origin',(26.5,28.5,0.));
#50313=CARTESIAN_POINT('',(25.,28.5,0.8));
#50314=CARTESIAN_POINT('',(25.,28.5,0.));
#50315=CARTESIAN_POINT('Origin',(26.5,28.5,0.8));
#50316=CARTESIAN_POINT('Origin',(25.,30.,0.));
#50317=CARTESIAN_POINT('',(25.,-28.5,0.8));
#50318=CARTESIAN_POINT('',(25.,-28.5,0.));
#50319=CARTESIAN_POINT('',(25.,15.,0.8));
#50320=CARTESIAN_POINT('Origin',(26.5,-28.5,0.));
#50321=CARTESIAN_POINT('',(26.5,-30.,0.8));
#50322=CARTESIAN_POINT('',(26.5,-30.,0.));
#50323=CARTESIAN_POINT('Origin',(26.5,-28.5,0.8));
#50324=CARTESIAN_POINT('Origin',(33.75,0.,0.));
#50325=CARTESIAN_POINT('',(38.5,-25.5,0.));
#50326=CARTESIAN_POINT('Origin',(39.5,-25.5,0.));
#50327=CARTESIAN_POINT('',(38.5,25.5,0.));
#50328=CARTESIAN_POINT('Origin',(39.5,25.5,0.));
#50329=CARTESIAN_POINT('Origin',(26.,4.8,1.));
#50330=CARTESIAN_POINT('',(26.,4.7,1.));
#50331=CARTESIAN_POINT('',(26.,4.7,1.));
#50332=CARTESIAN_POINT('',(26.,2.4,1.));
#50333=CARTESIAN_POINT('Origin',(34.,4.,1.));
#50334=CARTESIAN_POINT('',(34.,4.7,1.));
#50335=CARTESIAN_POINT('',(34.,2.,1.));
#50336=CARTESIAN_POINT('',(34.,4.7,1.));
#50337=CARTESIAN_POINT('Origin',(26.05,4.75,1.));
#50338=CARTESIAN_POINT('',(26.1,4.8,29.9));
#50339=CARTESIAN_POINT('',(26.,4.7,30.));
#50340=CARTESIAN_POINT('',(26.1,4.8,1.));
#50341=CARTESIAN_POINT('',(26.1,4.8,1.));
#50342=CARTESIAN_POINT('',(26.7875,5.48750000000002,1.));
#50343=CARTESIAN_POINT('Origin',(32.,4.75,29.95));
#50344=CARTESIAN_POINT('',(32.,4.8,29.9));
#50345=CARTESIAN_POINT('Origin',(34.,4.8,1.));
#50346=CARTESIAN_POINT('',(33.9,4.8,29.9));
#50347=CARTESIAN_POINT('',(32.,4.8,29.9));
#50348=CARTESIAN_POINT('',(33.9,4.8,1.));
#50349=CARTESIAN_POINT('',(33.9,4.8,1.));
#50350=CARTESIAN_POINT('',(33.875,4.8,1.));
#50351=CARTESIAN_POINT('',(29.025,4.8,17.));
#50352=CARTESIAN_POINT('Origin',(30.,4.8,17.));
#50353=CARTESIAN_POINT('',(29.025,4.8,6.));
#50354=CARTESIAN_POINT('Origin',(30.,4.8,6.));
#50355=CARTESIAN_POINT('Origin',(33.95,4.75,1.));
#50356=CARTESIAN_POINT('',(35.0875,3.61249999999994,1.));
#50357=CARTESIAN_POINT('',(33.9,4.8,29.9));
#50358=CARTESIAN_POINT('Origin',(32.,4.75,29.95));
#50359=CARTESIAN_POINT('Origin',(33.95,-4.75,1.));
#50360=CARTESIAN_POINT('',(33.9,-4.8,29.9));
#50361=CARTESIAN_POINT('',(34.,-4.7,30.));
#50362=CARTESIAN_POINT('',(33.9,-4.8,1.));
#50363=CARTESIAN_POINT('',(33.9,-4.8,1.));
#50364=CARTESIAN_POINT('',(34.,-4.7,1.));
#50365=CARTESIAN_POINT('',(35.0875,-3.61250000000002,1.));
#50366=CARTESIAN_POINT('',(34.,-4.7,1.));
#50367=CARTESIAN_POINT('Origin',(28.,-4.75,29.95));
#50368=CARTESIAN_POINT('',(28.,-4.8,29.9));
#50369=CARTESIAN_POINT('Origin',(26.,-4.8,1.));
#50370=CARTESIAN_POINT('',(30.8,-4.8,8.25));
#50371=CARTESIAN_POINT('',(29.875,-4.8,1.));
#50372=CARTESIAN_POINT('',(29.025,-4.8,17.));
#50373=CARTESIAN_POINT('Origin',(30.,-4.8,17.));
#50374=CARTESIAN_POINT('',(29.025,-4.8,6.));
#50375=CARTESIAN_POINT('Origin',(30.,-4.8,6.));
#50376=CARTESIAN_POINT('Origin',(26.,-4.,1.));
#50377=CARTESIAN_POINT('',(26.,-4.1,1.));
#50378=CARTESIAN_POINT('',(26.,-4.1,1.));
#50379=CARTESIAN_POINT('',(26.,-2.,1.));
#50380=CARTESIAN_POINT('Origin',(26.05,-4.05,1.));
#50381=CARTESIAN_POINT('',(26.1,-4.,1.));
#50382=CARTESIAN_POINT('',(26.1,-4.,1.));
#50383=CARTESIAN_POINT('',(28.9875,-1.11250000000002,1.));
#50384=CARTESIAN_POINT('Origin',(34.,-4.8,1.));
#50385=CARTESIAN_POINT('',(34.,-2.4,1.));
#50386=CARTESIAN_POINT('Origin',(30.,-4.05,17.));
#50387=CARTESIAN_POINT('',(29.025,-4.,17.));
#50388=CARTESIAN_POINT('Origin',(30.,-4.,17.));
#50389=CARTESIAN_POINT('',(29.125,-4.1,17.));
#50390=CARTESIAN_POINT('',(29.075,-4.05,17.));
#50391=CARTESIAN_POINT('Origin',(30.,-4.1,17.));
#50392=CARTESIAN_POINT('Origin',(30.,0.,17.));
#50393=CARTESIAN_POINT('',(29.125,-4.7,17.));
#50394=CARTESIAN_POINT('Origin',(30.,-4.7,17.));
#50395=CARTESIAN_POINT('',(29.125,0.,17.));
#50396=CARTESIAN_POINT('Origin',(34.,-4.,1.));
#50397=CARTESIAN_POINT('',(33.875,-4.,1.));
#50398=CARTESIAN_POINT('',(29.025,-4.,6.));
#50399=CARTESIAN_POINT('Origin',(30.,-4.,6.));
#50400=CARTESIAN_POINT('Origin',(30.,-4.75,17.));
#50401=CARTESIAN_POINT('',(29.075,-4.75,17.));
#50402=CARTESIAN_POINT('Origin',(30.,4.75,17.));
#50403=CARTESIAN_POINT('',(29.125,4.7,17.));
#50404=CARTESIAN_POINT('',(29.075,4.75,17.));
#50405=CARTESIAN_POINT('Origin',(30.,4.7,17.));
#50406=CARTESIAN_POINT('Origin',(30.,0.,17.));
#50407=CARTESIAN_POINT('',(29.125,4.1,17.));
#50408=CARTESIAN_POINT('Origin',(30.,4.1,17.));
#50409=CARTESIAN_POINT('',(29.125,0.,17.));
#50410=CARTESIAN_POINT('Origin',(30.,4.05,17.));
#50411=CARTESIAN_POINT('',(29.025,4.,17.));
#50412=CARTESIAN_POINT('Origin',(30.,4.,17.));
#50413=CARTESIAN_POINT('',(29.075,4.05,17.));
#50414=CARTESIAN_POINT('Origin',(26.,4.,1.));
#50415=CARTESIAN_POINT('',(29.875,4.,1.));
#50416=CARTESIAN_POINT('',(29.025,4.,6.));
#50417=CARTESIAN_POINT('Origin',(30.,4.,6.));
#50418=CARTESIAN_POINT('Origin',(30.,-4.05,6.));
#50419=CARTESIAN_POINT('',(29.125,-4.1,6.));
#50420=CARTESIAN_POINT('',(29.075,-4.05,6.));
#50421=CARTESIAN_POINT('Origin',(30.,-4.1,6.));
#50422=CARTESIAN_POINT('Origin',(30.,0.,6.));
#50423=CARTESIAN_POINT('',(29.125,-4.7,6.));
#50424=CARTESIAN_POINT('Origin',(30.,-4.7,6.));
#50425=CARTESIAN_POINT('',(29.125,0.,6.));
#50426=CARTESIAN_POINT('Origin',(30.,-4.75,6.));
#50427=CARTESIAN_POINT('',(29.075,-4.75,6.));
#50428=CARTESIAN_POINT('Origin',(30.,4.75,6.));
#50429=CARTESIAN_POINT('',(29.125,4.7,6.));
#50430=CARTESIAN_POINT('',(29.075,4.75,6.));
#50431=CARTESIAN_POINT('Origin',(30.,4.7,6.));
#50432=CARTESIAN_POINT('Origin',(30.,0.,6.));
#50433=CARTESIAN_POINT('',(29.125,4.1,6.));
#50434=CARTESIAN_POINT('Origin',(30.,4.1,6.));
#50435=CARTESIAN_POINT('',(29.125,0.,6.));
#50436=CARTESIAN_POINT('Origin',(30.,4.05,6.));
#50437=CARTESIAN_POINT('',(29.075,4.05,6.));
#50438=CARTESIAN_POINT('Origin',(39.5,-25.5,0.05));
#50439=CARTESIAN_POINT('',(38.6,-25.5,0.1));
#50440=CARTESIAN_POINT('',(38.55,-25.5,0.05));
#50441=CARTESIAN_POINT('Origin',(39.5,-25.5,0.1));
#50442=CARTESIAN_POINT('Origin',(39.5,-25.5,0.));
#50443=CARTESIAN_POINT('',(38.6,-25.5,0.9));
#50444=CARTESIAN_POINT('',(38.6,-25.5,0.));
#50445=CARTESIAN_POINT('Origin',(39.5,-25.5,0.9));
#50446=CARTESIAN_POINT('Origin',(39.5,25.5,0.05));
#50447=CARTESIAN_POINT('',(38.6,25.5,0.1));
#50448=CARTESIAN_POINT('',(38.55,25.5,0.05));
#50449=CARTESIAN_POINT('Origin',(39.5,25.5,0.1));
#50450=CARTESIAN_POINT('Origin',(39.5,25.5,0.));
#50451=CARTESIAN_POINT('',(38.6,25.5,0.9));
#50452=CARTESIAN_POINT('',(38.6,25.5,0.));
#50453=CARTESIAN_POINT('Origin',(39.5,25.5,0.9));
#50454=CARTESIAN_POINT('Origin',(31.5625,-29.7853553390593,0.964644660940671));
#50455=CARTESIAN_POINT('',(26.5,-29.7,1.));
#50456=CARTESIAN_POINT('',(31.5625,-29.7,1.));
#50457=CARTESIAN_POINT('',(26.5,-29.8707106781187,0.929289321881342));
#50458=CARTESIAN_POINT('',(26.5,-29.7,1.));
#50459=CARTESIAN_POINT('',(31.5625,-29.8707106781187,0.929289321881342));
#50460=CARTESIAN_POINT('Origin',(26.5,-28.5,0.964644660940672));
#50461=CARTESIAN_POINT('',(25.3,-28.5,1.));
#50462=CARTESIAN_POINT('',(25.1292893218813,-28.5,0.929289321881344));
#50463=CARTESIAN_POINT('',(25.3,-28.5,1.));
#50464=CARTESIAN_POINT('Origin',(26.5,-28.5,0.929289321881344));
#50465=CARTESIAN_POINT('Origin',(26.5,-28.5,1.));
#50466=CARTESIAN_POINT('Origin',(25.2146446609407,7.5,0.964644660940672));
#50467=CARTESIAN_POINT('',(25.3,28.5,1.));
#50468=CARTESIAN_POINT('',(25.1292893218813,28.5,0.929289321881344));
#50469=CARTESIAN_POINT('',(25.3,28.5,1.));
#50470=CARTESIAN_POINT('',(25.1292893218813,7.5,0.929289321881344));
#50471=CARTESIAN_POINT('',(25.3,7.5,1.));
#50472=CARTESIAN_POINT('Origin',(26.5,28.5,0.964644660940672));
#50473=CARTESIAN_POINT('',(26.5,29.7,1.));
#50474=CARTESIAN_POINT('',(26.5,29.8707106781187,0.929289321881344));
#50475=CARTESIAN_POINT('',(26.5,29.7,1.));
#50476=CARTESIAN_POINT('Origin',(26.5,28.5,0.929289321881344));
#50477=CARTESIAN_POINT('Origin',(26.5,28.5,1.));
#50478=CARTESIAN_POINT('Origin',(35.9375,29.7853553390593,0.964644660940671));
#50479=CARTESIAN_POINT('',(35.9375,29.8707106781187,0.929289321881342));
#50480=CARTESIAN_POINT('',(35.9375,29.7,1.));
#50481=CARTESIAN_POINT('Origin',(33.75,0.,1.));
#50482=CARTESIAN_POINT('',(30.8,-29.7,1.));
#50483=CARTESIAN_POINT('',(30.8,-8.7,1.));
#50484=CARTESIAN_POINT('',(41.,-29.7,1.));
#50485=CARTESIAN_POINT('',(31.5625,-29.7,1.));
#50486=CARTESIAN_POINT('',(42.2,-28.5,1.));
#50487=CARTESIAN_POINT('Origin',(41.,-28.5,1.));
#50488=CARTESIAN_POINT('',(42.2,28.5,1.));
#50489=CARTESIAN_POINT('',(42.2,-7.5,1.));
#50490=CARTESIAN_POINT('',(41.,29.7,1.));
#50491=CARTESIAN_POINT('Origin',(41.,28.5,1.));
#50492=CARTESIAN_POINT('',(35.9375,29.7,1.));
#50493=CARTESIAN_POINT('',(38.5,-25.5,1.));
#50494=CARTESIAN_POINT('Origin',(39.5,-25.5,1.));
#50495=CARTESIAN_POINT('',(38.5,25.5,1.));
#50496=CARTESIAN_POINT('Origin',(39.5,25.5,1.));
#50497=CARTESIAN_POINT('Origin',(35.9375,29.7853553390593,0.964644660940671));
#50498=CARTESIAN_POINT('',(41.,29.8707106781187,0.929289321881343));
#50499=CARTESIAN_POINT('',(41.,29.7,1.));
#50500=CARTESIAN_POINT('',(35.9375,29.8707106781187,0.929289321881342));
#50501=CARTESIAN_POINT('Origin',(41.,28.5,0.964644660940673));
#50502=CARTESIAN_POINT('',(42.3707106781187,28.5,0.929289321881346));
#50503=CARTESIAN_POINT('',(42.2,28.5,1.));
#50504=CARTESIAN_POINT('Origin',(41.,28.5,0.929289321881346));
#50505=CARTESIAN_POINT('Origin',(42.2853553390593,-7.5,0.964644660940672));
#50506=CARTESIAN_POINT('',(42.3707106781187,-28.5,0.929289321881343));
#50507=CARTESIAN_POINT('',(42.2,-28.5,1.));
#50508=CARTESIAN_POINT('',(42.3707106781187,-7.5,0.929289321881343));
#50509=CARTESIAN_POINT('Origin',(41.,-28.5,0.964644660940673));
#50510=CARTESIAN_POINT('',(41.,-29.8707106781187,0.929289321881346));
#50511=CARTESIAN_POINT('',(41.,-29.7,1.));
#50512=CARTESIAN_POINT('Origin',(41.,-28.5,0.929289321881346));
#50513=CARTESIAN_POINT('Origin',(31.5625,-29.7853553390593,0.964644660940671));
#50514=CARTESIAN_POINT('',(30.8,-29.8707106781187,0.929289321881342));
#50515=CARTESIAN_POINT('',(30.8,-21.9300622355798,4.21841360081793));
#50516=CARTESIAN_POINT('',(31.5625,-29.8707106781187,0.929289321881342));
#50517=CARTESIAN_POINT('Origin',(39.5,25.5,0.95));
#50518=CARTESIAN_POINT('',(38.55,25.5,0.95));
#50519=CARTESIAN_POINT('Origin',(39.5,-25.5,0.95));
#50520=CARTESIAN_POINT('',(38.55,-25.5,0.95));
#50521=CARTESIAN_POINT('Origin',(30.,-4.8,30.));
#50522=CARTESIAN_POINT('',(30.,-30.,1.));
#50523=CARTESIAN_POINT('Origin',(30.,-30.,1.));
#50524=CARTESIAN_POINT('',(30.8,-29.8,1.));
#50525=CARTESIAN_POINT('',(29.375,-29.8,1.));
#50526=CARTESIAN_POINT('',(30.8,-24.,1.));
#50527=CARTESIAN_POINT('Origin',(30.8,-17.4,15.5));
#50528=CARTESIAN_POINT('',(30.8,-23.125,7.67500000000001));
#50529=CARTESIAN_POINT('Origin',(26.5,-28.5,0.9));
#50530=CARTESIAN_POINT('',(25.2,-28.5,1.));
#50531=CARTESIAN_POINT('',(26.5,-30.,0.8));
#50532=CARTESIAN_POINT('Origin',(25.1,15.,0.9));
#50533=CARTESIAN_POINT('',(25.2,28.5,1.));
#50534=CARTESIAN_POINT('Origin',(26.5,28.5,0.9));
#50535=CARTESIAN_POINT('',(26.5,29.8,1.));
#50536=CARTESIAN_POINT('Origin',(38.125,29.9,0.9));
#50537=CARTESIAN_POINT('',(41.,29.8,1.));
#50538=CARTESIAN_POINT('Origin',(41.,28.5,0.9));
#50539=CARTESIAN_POINT('',(42.5,28.5,0.8));
#50540=CARTESIAN_POINT('',(42.3,28.5,1.));
#50541=CARTESIAN_POINT('Origin',(41.,28.5,0.8));
#50542=CARTESIAN_POINT('Origin',(42.4,-15.,0.9));
#50543=CARTESIAN_POINT('',(42.5,-28.5,0.8));
#50544=CARTESIAN_POINT('',(42.3,-28.5,1.));
#50545=CARTESIAN_POINT('',(42.5,-15.,0.8));
#50546=CARTESIAN_POINT('Origin',(41.,-28.5,0.9));
#50547=CARTESIAN_POINT('',(41.,-30.,0.8));
#50548=CARTESIAN_POINT('',(41.,-29.8,1.));
#50549=CARTESIAN_POINT('Origin',(41.,-28.5,0.8));
#50550=CARTESIAN_POINT('Origin',(29.375,-29.9,0.9));
#50551=CARTESIAN_POINT('',(29.375,-30.,0.8));
#50552=CARTESIAN_POINT('Origin',(42.5,-30.,0.));
#50553=CARTESIAN_POINT('',(42.5,28.5,0.));
#50554=CARTESIAN_POINT('',(42.5,-28.5,0.));
#50555=CARTESIAN_POINT('Origin',(41.,-28.5,0.));
#50556=CARTESIAN_POINT('',(41.,-30.,0.));
#50557=CARTESIAN_POINT('Origin',(25.,-30.,0.));
#50558=CARTESIAN_POINT('Origin',(41.,28.5,0.));
#71462=UNCERTAINTY_MEASURE_WITH_UNIT(LENGTH_MEASURE(0.001),#71493,
'DISTANCE_ACCURACY_VALUE',
'Maximum model space distance between geometric entities at asserted c
onnectivities');
#71471=UNCERTAINTY_MEASURE_WITH_UNIT(LENGTH_MEASURE(0.001),#71493,
'DISTANCE_ACCURACY_VALUE',
'Maximum model space distance between geometric entities at asserted c
onnectivities');
#71483=(
GEOMETRIC_REPRESENTATION_CONTEXT(3)
GLOBAL_UNCERTAINTY_ASSIGNED_CONTEXT((#71462))
GLOBAL_UNIT_ASSIGNED_CONTEXT((#71493,#71495,#71496))
REPRESENTATION_CONTEXT('','3D')
);
#71492=(
GEOMETRIC_REPRESENTATION_CONTEXT(3)
GLOBAL_UNCERTAINTY_ASSIGNED_CONTEXT((#71471))
GLOBAL_UNIT_ASSIGNED_CONTEXT((#71493,#71495,#71496))
REPRESENTATION_CONTEXT('','3D')
);
#71493=(
LENGTH_UNIT()
NAMED_UNIT(*)
SI_UNIT(.CENTI.,.METRE.)
);
#71495=(
NAMED_UNIT(*)
PLANE_ANGLE_UNIT()
SI_UNIT($,.RADIAN.)
);
#71496=(
NAMED_UNIT(*)
SI_UNIT($,.STERADIAN.)
SOLID_ANGLE_UNIT()
);
#71508=SHAPE_DEFINITION_REPRESENTATION(#71528,#71613);
#71528=PRODUCT_DEFINITION_SHAPE('',$,#71634);
#71613=SHAPE_REPRESENTATION('',(#30013),#71483);
#71622=PRODUCT_DEFINITION_CONTEXT('part definition',#71684,'design');
#71634=PRODUCT_DEFINITION('2026-10-19-03-21-55-709',
'07_Frame_Base_Anchor_Plate_600x175_Foot',#71654,#71622);
#71654=PRODUCT_DEFINITION_FORMATION('',$,#71697);
#71684=APPLICATION_CONTEXT(
'Core Data for Automotive Mechanical Design Process');
#71685=PRODUCT_CONTEXT('part definition',#71684,'mechanical');
#71697=PRODUCT('2026-10-19-03-21-55-709',
'07_Frame_Base_Anchor_Plate_600x175_Foot',$,(#71685));
#71860=COLOUR_RGB('Dark Blue',0.08,0.2,0.34);
#71861=FILL_AREA_STYLE_COLOUR('',#71860);
#71862=FILL_AREA_STYLE('',(#71861));
#71863=SURFACE_STYLE_FILL_AREA(#71862);
#71864=SURFACE_SIDE_STYLE('',(#71863));
#71865=SURFACE_STYLE_USAGE(.BOTH.,#71864);
#71866=PRESENTATION_STYLE_ASSIGNMENT((#71865));
ENDSEC;
END-ISO-10303-21;
